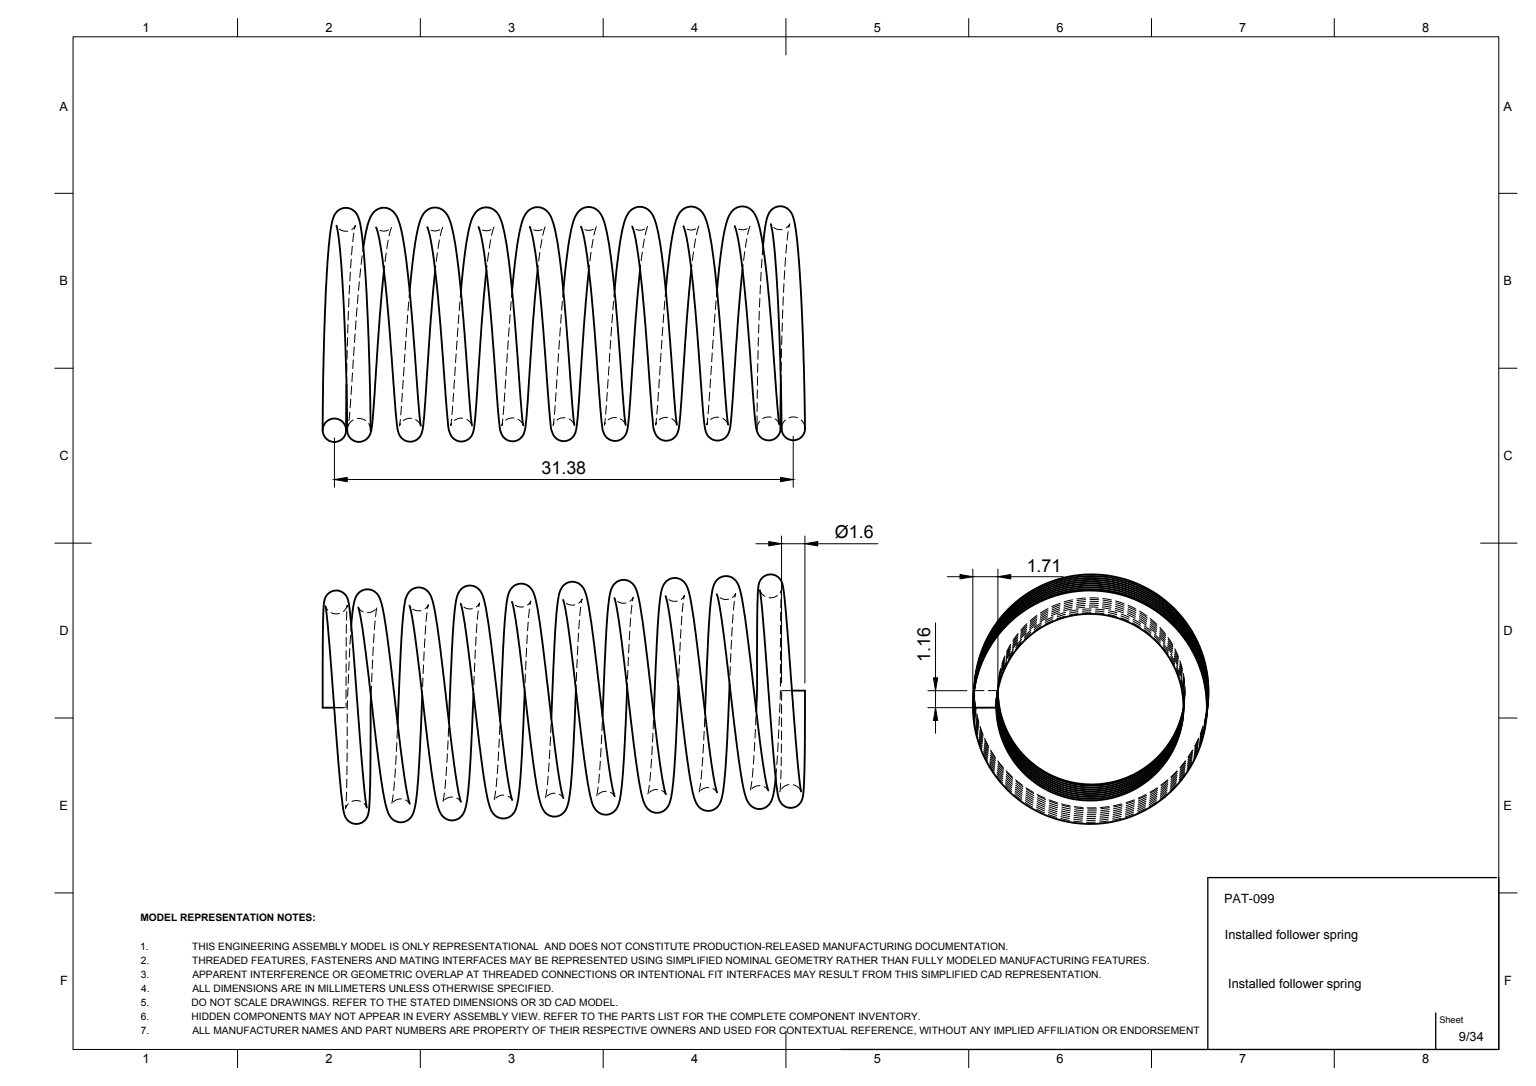
ISO-10303-21;
HEADER;
/* Generated by software containing ST-Developer
 * from STEP Tools, Inc. (www.steptools.com) 
 */

FILE_DESCRIPTION(
/* description */ ('PAT-099'),
/* implementation_level */ '2;1');

FILE_NAME(
/* name */ 'Installed follower spring.step',
/* time_stamp */ '2026-10-29T17:25:42-07:00',
/* author */ (''),
/* organization */ (''),
/* preprocessor_version */ 'ST-DEVELOPER v20.2',
/* originating_system */ 'Autodesk Translation Framework v15.17.0.0',
/* authorisation */ '');

FILE_SCHEMA (('AUTOMOTIVE_DESIGN { 1 0 10303 214 3 1 1 }'));
ENDSEC;

DATA;
#10=MECHANICAL_DESIGN_GEOMETRIC_PRESENTATION_REPRESENTATION('',(#341),#11035);
#240=B_SPLINE_SURFACE_WITH_KNOTS('',3,3,((#7917,#7918,#7919,#7920,#7921,
#7922,#7923,#7924,#7925,#7926,#7927,#7928,#7929,#7930,#7931,#7932,#7933,
#7934,#7935,#7936,#7937,#7938,#7939,#7940,#7941,#7942,#7943,#7944,#7945,
#7946,#7947,#7948,#7949,#7950,#7951,#7952,#7953,#7954,#7955,#7956,#7957,
#7958,#7959,#7960,#7961,#7962,#7963,#7964,#7965,#7966,#7967,#7968,#7969,
#7970,#7971,#7972,#7973,#7974,#7975,#7976,#7977,#7978,#7979,#7980,#7981,
#7982,#7983,#7984,#7985,#7986,#7987,#7988,#7989,#7990,#7991,#7992,#7993,
#7994,#7995,#7996,#7997,#7998,#7999,#8000,#8001,#8002,#8003,#8004,#8005,
#8006,#8007,#8008,#8009,#8010,#8011,#8012,#8013,#8014,#8015,#8016,#8017,
#8018,#8019,#8020,#8021,#8022,#8023,#8024,#8025,#8026,#8027,#8028,#8029,
#8030,#8031,#8032,#8033,#8034,#8035,#8036,#8037,#8038,#8039,#8040,#8041,
#8042,#8043,#8044,#8045,#8046,#8047,#8048,#8049,#8050,#8051,#8052,#8053,
#8054,#8055,#8056),(#8057,#8058,#8059,#8060,#8061,#8062,#8063,#8064,#8065,
#8066,#8067,#8068,#8069,#8070,#8071,#8072,#8073,#8074,#8075,#8076,#8077,
#8078,#8079,#8080,#8081,#8082,#8083,#8084,#8085,#8086,#8087,#8088,#8089,
#8090,#8091,#8092,#8093,#8094,#8095,#8096,#8097,#8098,#8099,#8100,#8101,
#8102,#8103,#8104,#8105,#8106,#8107,#8108,#8109,#8110,#8111,#8112,#8113,
#8114,#8115,#8116,#8117,#8118,#8119,#8120,#8121,#8122,#8123,#8124,#8125,
#8126,#8127,#8128,#8129,#8130,#8131,#8132,#8133,#8134,#8135,#8136,#8137,
#8138,#8139,#8140,#8141,#8142,#8143,#8144,#8145,#8146,#8147,#8148,#8149,
#8150,#8151,#8152,#8153,#8154,#8155,#8156,#8157,#8158,#8159,#8160,#8161,
#8162,#8163,#8164,#8165,#8166,#8167,#8168,#8169,#8170,#8171,#8172,#8173,
#8174,#8175,#8176,#8177,#8178,#8179,#8180,#8181,#8182,#8183,#8184,#8185,
#8186,#8187,#8188,#8189,#8190,#8191,#8192,#8193,#8194,#8195,#8196),(#8197,
#8198,#8199,#8200,#8201,#8202,#8203,#8204,#8205,#8206,#8207,#8208,#8209,
#8210,#8211,#8212,#8213,#8214,#8215,#8216,#8217,#8218,#8219,#8220,#8221,
#8222,#8223,#8224,#8225,#8226,#8227,#8228,#8229,#8230,#8231,#8232,#8233,
#8234,#8235,#8236,#8237,#8238,#8239,#8240,#8241,#8242,#8243,#8244,#8245,
#8246,#8247,#8248,#8249,#8250,#8251,#8252,#8253,#8254,#8255,#8256,#8257,
#8258,#8259,#8260,#8261,#8262,#8263,#8264,#8265,#8266,#8267,#8268,#8269,
#8270,#8271,#8272,#8273,#8274,#8275,#8276,#8277,#8278,#8279,#8280,#8281,
#8282,#8283,#8284,#8285,#8286,#8287,#8288,#8289,#8290,#8291,#8292,#8293,
#8294,#8295,#8296,#8297,#8298,#8299,#8300,#8301,#8302,#8303,#8304,#8305,
#8306,#8307,#8308,#8309,#8310,#8311,#8312,#8313,#8314,#8315,#8316,#8317,
#8318,#8319,#8320,#8321,#8322,#8323,#8324,#8325,#8326,#8327,#8328,#8329,
#8330,#8331,#8332,#8333,#8334,#8335,#8336),(#8337,#8338,#8339,#8340,#8341,
#8342,#8343,#8344,#8345,#8346,#8347,#8348,#8349,#8350,#8351,#8352,#8353,
#8354,#8355,#8356,#8357,#8358,#8359,#8360,#8361,#8362,#8363,#8364,#8365,
#8366,#8367,#8368,#8369,#8370,#8371,#8372,#8373,#8374,#8375,#8376,#8377,
#8378,#8379,#8380,#8381,#8382,#8383,#8384,#8385,#8386,#8387,#8388,#8389,
#8390,#8391,#8392,#8393,#8394,#8395,#8396,#8397,#8398,#8399,#8400,#8401,
#8402,#8403,#8404,#8405,#8406,#8407,#8408,#8409,#8410,#8411,#8412,#8413,
#8414,#8415,#8416,#8417,#8418,#8419,#8420,#8421,#8422,#8423,#8424,#8425,
#8426,#8427,#8428,#8429,#8430,#8431,#8432,#8433,#8434,#8435,#8436,#8437,
#8438,#8439,#8440,#8441,#8442,#8443,#8444,#8445,#8446,#8447,#8448,#8449,
#8450,#8451,#8452,#8453,#8454,#8455,#8456,#8457,#8458,#8459,#8460,#8461,
#8462,#8463,#8464,#8465,#8466,#8467,#8468,#8469,#8470,#8471,#8472,#8473,
#8474,#8475,#8476),(#8477,#8478,#8479,#8480,#8481,#8482,#8483,#8484,#8485,
#8486,#8487,#8488,#8489,#8490,#8491,#8492,#8493,#8494,#8495,#8496,#8497,
#8498,#8499,#8500,#8501,#8502,#8503,#8504,#8505,#8506,#8507,#8508,#8509,
#8510,#8511,#8512,#8513,#8514,#8515,#8516,#8517,#8518,#8519,#8520,#8521,
#8522,#8523,#8524,#8525,#8526,#8527,#8528,#8529,#8530,#8531,#8532,#8533,
#8534,#8535,#8536,#8537,#8538,#8539,#8540,#8541,#8542,#8543,#8544,#8545,
#8546,#8547,#8548,#8549,#8550,#8551,#8552,#8553,#8554,#8555,#8556,#8557,
#8558,#8559,#8560,#8561,#8562,#8563,#8564,#8565,#8566,#8567,#8568,#8569,
#8570,#8571,#8572,#8573,#8574,#8575,#8576,#8577,#8578,#8579,#8580,#8581,
#8582,#8583,#8584,#8585,#8586,#8587,#8588,#8589,#8590,#8591,#8592,#8593,
#8594,#8595,#8596,#8597,#8598,#8599,#8600,#8601,#8602,#8603,#8604,#8605,
#8606,#8607,#8608,#8609,#8610,#8611,#8612,#8613,#8614,#8615,#8616),(#8617,
#8618,#8619,#8620,#8621,#8622,#8623,#8624,#8625,#8626,#8627,#8628,#8629,
#8630,#8631,#8632,#8633,#8634,#8635,#8636,#8637,#8638,#8639,#8640,#8641,
#8642,#8643,#8644,#8645,#8646,#8647,#8648,#8649,#8650,#8651,#8652,#8653,
#8654,#8655,#8656,#8657,#8658,#8659,#8660,#8661,#8662,#8663,#8664,#8665,
#8666,#8667,#8668,#8669,#8670,#8671,#8672,#8673,#8674,#8675,#8676,#8677,
#8678,#8679,#8680,#8681,#8682,#8683,#8684,#8685,#8686,#8687,#8688,#8689,
#8690,#8691,#8692,#8693,#8694,#8695,#8696,#8697,#8698,#8699,#8700,#8701,
#8702,#8703,#8704,#8705,#8706,#8707,#8708,#8709,#8710,#8711,#8712,#8713,
#8714,#8715,#8716,#8717,#8718,#8719,#8720,#8721,#8722,#8723,#8724,#8725,
#8726,#8727,#8728,#8729,#8730,#8731,#8732,#8733,#8734,#8735,#8736,#8737,
#8738,#8739,#8740,#8741,#8742,#8743,#8744,#8745,#8746,#8747,#8748,#8749,
#8750,#8751,#8752,#8753,#8754,#8755,#8756),(#8757,#8758,#8759,#8760,#8761,
#8762,#8763,#8764,#8765,#8766,#8767,#8768,#8769,#8770,#8771,#8772,#8773,
#8774,#8775,#8776,#8777,#8778,#8779,#8780,#8781,#8782,#8783,#8784,#8785,
#8786,#8787,#8788,#8789,#8790,#8791,#8792,#8793,#8794,#8795,#8796,#8797,
#8798,#8799,#8800,#8801,#8802,#8803,#8804,#8805,#8806,#8807,#8808,#8809,
#8810,#8811,#8812,#8813,#8814,#8815,#8816,#8817,#8818,#8819,#8820,#8821,
#8822,#8823,#8824,#8825,#8826,#8827,#8828,#8829,#8830,#8831,#8832,#8833,
#8834,#8835,#8836,#8837,#8838,#8839,#8840,#8841,#8842,#8843,#8844,#8845,
#8846,#8847,#8848,#8849,#8850,#8851,#8852,#8853,#8854,#8855,#8856,#8857,
#8858,#8859,#8860,#8861,#8862,#8863,#8864,#8865,#8866,#8867,#8868,#8869,
#8870,#8871,#8872,#8873,#8874,#8875,#8876,#8877,#8878,#8879,#8880,#8881,
#8882,#8883,#8884,#8885,#8886,#8887,#8888,#8889,#8890,#8891,#8892,#8893,
#8894,#8895,#8896),(#8897,#8898,#8899,#8900,#8901,#8902,#8903,#8904,#8905,
#8906,#8907,#8908,#8909,#8910,#8911,#8912,#8913,#8914,#8915,#8916,#8917,
#8918,#8919,#8920,#8921,#8922,#8923,#8924,#8925,#8926,#8927,#8928,#8929,
#8930,#8931,#8932,#8933,#8934,#8935,#8936,#8937,#8938,#8939,#8940,#8941,
#8942,#8943,#8944,#8945,#8946,#8947,#8948,#8949,#8950,#8951,#8952,#8953,
#8954,#8955,#8956,#8957,#8958,#8959,#8960,#8961,#8962,#8963,#8964,#8965,
#8966,#8967,#8968,#8969,#8970,#8971,#8972,#8973,#8974,#8975,#8976,#8977,
#8978,#8979,#8980,#8981,#8982,#8983,#8984,#8985,#8986,#8987,#8988,#8989,
#8990,#8991,#8992,#8993,#8994,#8995,#8996,#8997,#8998,#8999,#9000,#9001,
#9002,#9003,#9004,#9005,#9006,#9007,#9008,#9009,#9010,#9011,#9012,#9013,
#9014,#9015,#9016,#9017,#9018,#9019,#9020,#9021,#9022,#9023,#9024,#9025,
#9026,#9027,#9028,#9029,#9030,#9031,#9032,#9033,#9034,#9035,#9036),(#9037,
#9038,#9039,#9040,#9041,#9042,#9043,#9044,#9045,#9046,#9047,#9048,#9049,
#9050,#9051,#9052,#9053,#9054,#9055,#9056,#9057,#9058,#9059,#9060,#9061,
#9062,#9063,#9064,#9065,#9066,#9067,#9068,#9069,#9070,#9071,#9072,#9073,
#9074,#9075,#9076,#9077,#9078,#9079,#9080,#9081,#9082,#9083,#9084,#9085,
#9086,#9087,#9088,#9089,#9090,#9091,#9092,#9093,#9094,#9095,#9096,#9097,
#9098,#9099,#9100,#9101,#9102,#9103,#9104,#9105,#9106,#9107,#9108,#9109,
#9110,#9111,#9112,#9113,#9114,#9115,#9116,#9117,#9118,#9119,#9120,#9121,
#9122,#9123,#9124,#9125,#9126,#9127,#9128,#9129,#9130,#9131,#9132,#9133,
#9134,#9135,#9136,#9137,#9138,#9139,#9140,#9141,#9142,#9143,#9144,#9145,
#9146,#9147,#9148,#9149,#9150,#9151,#9152,#9153,#9154,#9155,#9156,#9157,
#9158,#9159,#9160,#9161,#9162,#9163,#9164,#9165,#9166,#9167,#9168,#9169,
#9170,#9171,#9172,#9173,#9174,#9175,#9176),(#9177,#9178,#9179,#9180,#9181,
#9182,#9183,#9184,#9185,#9186,#9187,#9188,#9189,#9190,#9191,#9192,#9193,
#9194,#9195,#9196,#9197,#9198,#9199,#9200,#9201,#9202,#9203,#9204,#9205,
#9206,#9207,#9208,#9209,#9210,#9211,#9212,#9213,#9214,#9215,#9216,#9217,
#9218,#9219,#9220,#9221,#9222,#9223,#9224,#9225,#9226,#9227,#9228,#9229,
#9230,#9231,#9232,#9233,#9234,#9235,#9236,#9237,#9238,#9239,#9240,#9241,
#9242,#9243,#9244,#9245,#9246,#9247,#9248,#9249,#9250,#9251,#9252,#9253,
#9254,#9255,#9256,#9257,#9258,#9259,#9260,#9261,#9262,#9263,#9264,#9265,
#9266,#9267,#9268,#9269,#9270,#9271,#9272,#9273,#9274,#9275,#9276,#9277,
#9278,#9279,#9280,#9281,#9282,#9283,#9284,#9285,#9286,#9287,#9288,#9289,
#9290,#9291,#9292,#9293,#9294,#9295,#9296,#9297,#9298,#9299,#9300,#9301,
#9302,#9303,#9304,#9305,#9306,#9307,#9308,#9309,#9310,#9311,#9312,#9313,
#9314,#9315,#9316)),.UNSPECIFIED.,.T.,.F.,.F.,(4,1,1,1,1,1,1,4),(4,1,1,
1,1,1,1,1,1,1,1,1,1,1,1,1,1,1,1,1,1,1,1,1,1,1,1,1,1,1,1,1,1,1,1,1,1,1,1,
1,1,1,1,1,1,1,1,1,1,1,1,1,1,1,1,1,1,1,1,1,1,1,1,1,1,1,1,1,1,1,1,1,1,1,1,
1,1,1,1,1,1,1,1,1,1,1,1,1,1,1,1,1,1,1,1,1,1,1,1,1,1,1,1,1,1,1,1,1,1,1,1,
1,1,1,1,1,1,1,1,1,1,1,1,1,1,1,1,1,1,1,1,1,1,1,1,1,1,4),(-3.14159265358979,
-2.24399475256414,-1.34639685153848,-0.448798950512828,0.448798950512828,
1.34639685153848,2.24399475256414,3.14159265358979),(0.,0.00892857142857143,
0.0178571428571429,0.0267857142857143,0.0357142857142857,0.0446428571428571,
0.0535714285714286,0.0625,0.0714285714285714,0.0758928571428571,0.0803571428571428,
0.0848214285714286,0.0892857142857143,0.09375,0.0948660714285714,0.0959821428571428,
0.0970982142857143,0.0982142857142857,0.100446428571429,0.102678571428571,
0.107142857142857,0.116071428571429,0.120535714285714,0.125,0.133928571428571,
0.142857142857143,0.150793650793651,0.158730158730159,0.166666666666667,
0.174603174603175,0.182539682539683,0.19047619047619,0.196428571428571,
0.202380952380952,0.214285714285714,0.222222222222222,0.23015873015873,
0.238095238095238,0.241071428571429,0.244047619047619,0.25,0.261904761904762,
0.273809523809524,0.285714285714286,0.297619047619048,0.30952380952381,
0.321428571428571,0.327380952380952,0.333333333333333,0.341269841269841,
0.349206349206349,0.357142857142857,0.361111111111111,0.365079365079365,
0.373015873015873,0.380952380952381,0.392857142857143,0.398809523809524,
0.404761904761905,0.416666666666667,0.428571428571429,0.4375,0.446428571428571,
0.455357142857143,0.457589285714286,0.459821428571429,0.462053571428571,
0.464285714285714,0.470238095238095,0.482142857142857,0.491071428571429,
0.5,0.508928571428571,0.517857142857143,0.526785714285714,0.535714285714286,
0.544642857142857,0.553571428571429,0.5625,0.571428571428571,0.580357142857143,
0.589285714285714,0.598214285714286,0.607142857142857,0.616071428571429,
0.625,0.633928571428571,0.638392857142857,0.642857142857143,0.650793650793651,
0.658730158730159,0.666666666666667,0.672619047619048,0.678571428571428,
0.69047619047619,0.702380952380952,0.714285714285714,0.726190476190476,
0.738095238095238,0.744047619047619,0.75,0.761904761904762,0.76984126984127,
0.777777777777778,0.785714285714286,0.794642857142857,0.803571428571428,
0.8125,0.821428571428571,0.830357142857143,0.839285714285714,0.848214285714286,
0.857142857142857,0.866071428571429,0.875,0.879464285714286,0.883928571428571,
0.892857142857143,0.897321428571428,0.899553571428571,0.901785714285714,
0.902901785714286,0.904017857142857,0.905133928571429,0.90625,0.910714285714286,
0.915178571428571,0.919642857142857,0.924107142857143,0.928571428571429,
0.9375,0.946428571428571,0.955357142857143,0.964285714285714,0.973214285714286,
0.982142857142857,0.991071428571429,1.),.UNSPECIFIED.);
#259=B_SPLINE_CURVE_WITH_KNOTS('',3,(#9320,#9321,#9322,#9323,#9324,#9325,
#9326,#9327,#9328,#9329,#9330,#9331,#9332,#9333,#9334,#9335,#9336,#9337,
#9338,#9339,#9340,#9341,#9342,#9343,#9344,#9345,#9346,#9347,#9348,#9349,
#9350,#9351,#9352,#9353,#9354,#9355,#9356,#9357,#9358,#9359,#9360,#9361,
#9362,#9363,#9364,#9365,#9366,#9367,#9368,#9369,#9370,#9371,#9372,#9373,
#9374,#9375,#9376,#9377,#9378,#9379,#9380,#9381,#9382,#9383,#9384,#9385,
#9386,#9387,#9388,#9389,#9390,#9391,#9392,#9393,#9394,#9395,#9396,#9397,
#9398,#9399,#9400,#9401,#9402,#9403,#9404,#9405,#9406,#9407,#9408,#9409,
#9410,#9411,#9412,#9413,#9414,#9415,#9416,#9417,#9418,#9419,#9420,#9421,
#9422,#9423,#9424,#9425,#9426,#9427,#9428,#9429,#9430,#9431,#9432,#9433,
#9434,#9435,#9436,#9437,#9438,#9439,#9440,#9441,#9442,#9443,#9444,#9445,
#9446,#9447,#9448,#9449,#9450,#9451,#9452,#9453,#9454,#9455,#9456,#9457,
#9458,#9459),.UNSPECIFIED.,.F.,.F.,(4,1,1,1,1,1,1,1,1,1,1,1,1,1,1,1,1,1,
1,1,1,1,1,1,1,1,1,1,1,1,1,1,1,1,1,1,1,1,1,1,1,1,1,1,1,1,1,1,1,1,1,1,1,1,
1,1,1,1,1,1,1,1,1,1,1,1,1,1,1,1,1,1,1,1,1,1,1,1,1,1,1,1,1,1,1,1,1,1,1,1,
1,1,1,1,1,1,1,1,1,1,1,1,1,1,1,1,1,1,1,1,1,1,1,1,1,1,1,1,1,1,1,1,1,1,1,1,
1,1,1,1,1,1,1,1,1,1,1,4),(0.,0.00892857142857143,0.0178571428571429,0.0267857142857143,
0.0357142857142857,0.0446428571428571,0.0535714285714286,0.0625,0.0714285714285714,
0.0758928571428571,0.0803571428571428,0.0848214285714286,0.0892857142857143,
0.09375,0.0948660714285714,0.0959821428571428,0.0970982142857143,0.0982142857142857,
0.100446428571429,0.102678571428571,0.107142857142857,0.116071428571429,
0.120535714285714,0.125,0.133928571428571,0.142857142857143,0.150793650793651,
0.158730158730159,0.166666666666667,0.174603174603175,0.182539682539683,
0.19047619047619,0.196428571428571,0.202380952380952,0.214285714285714,
0.222222222222222,0.23015873015873,0.238095238095238,0.241071428571429,
0.244047619047619,0.25,0.261904761904762,0.273809523809524,0.285714285714286,
0.297619047619048,0.30952380952381,0.321428571428571,0.327380952380952,
0.333333333333333,0.341269841269841,0.349206349206349,0.357142857142857,
0.361111111111111,0.365079365079365,0.373015873015873,0.380952380952381,
0.392857142857143,0.398809523809524,0.404761904761905,0.416666666666667,
0.428571428571429,0.4375,0.446428571428571,0.455357142857143,0.457589285714286,
0.459821428571429,0.462053571428571,0.464285714285714,0.470238095238095,
0.482142857142857,0.491071428571429,0.5,0.508928571428571,0.517857142857143,
0.526785714285714,0.535714285714286,0.544642857142857,0.553571428571429,
0.5625,0.571428571428571,0.580357142857143,0.589285714285714,0.598214285714286,
0.607142857142857,0.616071428571429,0.625,0.633928571428571,0.638392857142857,
0.642857142857143,0.650793650793651,0.658730158730159,0.666666666666667,
0.672619047619048,0.678571428571428,0.69047619047619,0.702380952380952,
0.714285714285714,0.726190476190476,0.738095238095238,0.744047619047619,
0.75,0.761904761904762,0.76984126984127,0.777777777777778,0.785714285714286,
0.794642857142857,0.803571428571428,0.8125,0.821428571428571,0.830357142857143,
0.839285714285714,0.848214285714286,0.857142857142857,0.866071428571429,
0.875,0.879464285714286,0.883928571428571,0.892857142857143,0.897321428571428,
0.899553571428571,0.901785714285714,0.902901785714286,0.904017857142857,
0.905133928571429,0.90625,0.910714285714286,0.915178571428571,0.919642857142857,
0.924107142857143,0.928571428571429,0.9375,0.946428571428571,0.955357142857143,
0.964285714285714,0.973214285714286,0.982142857142857,0.991071428571429,
1.),.UNSPECIFIED.);
#291=SHAPE_REPRESENTATION_RELATIONSHIP('SRR','None',#11159,#316);
#316=ADVANCED_BREP_SHAPE_REPRESENTATION('',(#374),#11009);
#341=STYLED_ITEM('',(#11386),#374);
#374=MANIFOLD_SOLID_BREP('Body1',#4709);
#541=PLANE('',#5146);
#542=PLANE('',#5147);
#714=FACE_OUTER_BOUND('',#1039,.T.);
#715=FACE_OUTER_BOUND('',#1040,.T.);
#716=FACE_OUTER_BOUND('',#1041,.T.);
#1039=EDGE_LOOP('',(#3421,#3422,#3423,#3424));
#1040=EDGE_LOOP('',(#3425));
#1041=EDGE_LOOP('',(#3426));
#1913=CIRCLE('',#5144,0.08);
#1914=CIRCLE('',#5145,0.08);
#2238=VERTEX_POINT('',#9317);
#2239=VERTEX_POINT('',#9319);
#2687=EDGE_CURVE('',#2238,#2238,#1913,.T.);
#2688=EDGE_CURVE('',#2238,#2239,#259,.T.);
#2689=EDGE_CURVE('',#2239,#2239,#1914,.T.);
#3421=ORIENTED_EDGE('',*,*,#2687,.T.);
#3422=ORIENTED_EDGE('',*,*,#2688,.T.);
#3423=ORIENTED_EDGE('',*,*,#2689,.F.);
#3424=ORIENTED_EDGE('',*,*,#2688,.F.);
#3425=ORIENTED_EDGE('',*,*,#2689,.T.);
#3426=ORIENTED_EDGE('',*,*,#2687,.F.);
#4479=ADVANCED_FACE('',(#714),#240,.T.);
#4480=ADVANCED_FACE('',(#715),#541,.T.);
#4481=ADVANCED_FACE('',(#716),#542,.F.);
#4709=CLOSED_SHELL('',(#4479,#4480,#4481));
#5143=AXIS2_PLACEMENT_3D('',#7916,#5983,#5984);
#5144=AXIS2_PLACEMENT_3D('',#9318,#5985,#5986);
#5145=AXIS2_PLACEMENT_3D('',#9460,#5987,#5988);
#5146=AXIS2_PLACEMENT_3D('',#9461,#5989,#5990);
#5147=AXIS2_PLACEMENT_3D('',#9462,#5991,#5992);
#5983=DIRECTION('axis',(0.,0.,1.));
#5984=DIRECTION('refdir',(1.,0.,0.));
#5985=DIRECTION('center_axis',(0.0370000185832032,-0.000134528644531496,
0.999315255826152));
#5986=DIRECTION('ref_axis',(-0.999308650506119,0.00363339380273223,0.0370002631492478));
#5987=DIRECTION('center_axis',(0.0370000189191082,0.000134528641494255,
0.999315255813715));
#5988=DIRECTION('ref_axis',(0.351666218592536,-0.936036645094244,-0.0128945624795743));
#5989=DIRECTION('center_axis',(0.0370000189191082,0.000134528641494255,
0.999315255813715));
#5990=DIRECTION('ref_axis',(0.351666218592536,-0.936036645094244,-0.0128945624795743));
#5991=DIRECTION('center_axis',(0.0370000185832032,-0.000134528644531496,
0.999315255826152));
#5992=DIRECTION('ref_axis',(-0.999308650506119,0.00363339380273222,0.0370002631492478));
#7916=CARTESIAN_POINT('',(0.,0.,0.));
#7917=CARTESIAN_POINT('Ctrl Pts',(6.55994469204049,0.719709328495781,5.24703997894806));
#7918=CARTESIAN_POINT('Ctrl Pts',(6.56494552765653,0.719691145920131,5.38210508200347));
#7919=CARTESIAN_POINT('Ctrl Pts',(6.57494016333875,0.642089168505731,5.65058609468785));
#7920=CARTESIAN_POINT('Ctrl Pts',(6.58989438616266,0.32941528595114,5.9296313569664));
#7921=CARTESIAN_POINT('Ctrl Pts',(6.60481477071411,-0.0827797453005289,
5.99886361370576));
#7922=CARTESIAN_POINT('Ctrl Pts',(6.61969980345594,-0.467619845512657,5.83844773036597));
#7923=CARTESIAN_POINT('Ctrl Pts',(6.63454965842308,-0.707639327219362,5.49857002500469));
#7924=CARTESIAN_POINT('Ctrl Pts',(6.64936061260475,-0.729495436544756,5.0840660001111));
#7925=CARTESIAN_POINT('Ctrl Pts',(6.66414030226907,-0.527844751315962,4.72224444577032));
#7926=CARTESIAN_POINT('Ctrl Pts',(6.67641810037933,-0.225796647591973,4.55722222010489));
#7927=CARTESIAN_POINT('Ctrl Pts',(6.68623494447203,0.0403746271135037,4.5362580751361));
#7928=CARTESIAN_POINT('Ctrl Pts',(6.69357256905876,0.236291461979514,4.57606849800983));
#7929=CARTESIAN_POINT('Ctrl Pts',(6.70093718034598,0.413303779793928,4.66864974641035));
#7930=CARTESIAN_POINT('Ctrl Pts',(6.70820868996388,0.557592736564421,4.80642809587619));
#7931=CARTESIAN_POINT('Ctrl Pts',(6.71380490830661,0.632807795501951,4.93556873282767));
#7932=CARTESIAN_POINT('Ctrl Pts',(6.71731244248601,0.666836920456702,5.02812885948168));
#7933=CARTESIAN_POINT('Ctrl Pts',(6.71917582310349,0.680406120596861,5.07513188532028));
#7934=CARTESIAN_POINT('Ctrl Pts',(6.72133213271133,0.6909093875254,5.1233938812218));
#7935=CARTESIAN_POINT('Ctrl Pts',(6.72306773259333,0.700241175081311,5.19054637990825));
#7936=CARTESIAN_POINT('Ctrl Pts',(6.72619261442483,0.703178325652587,5.2668476785023));
#7937=CARTESIAN_POINT('Ctrl Pts',(6.7381664251681,0.689514001675121,5.39852659753196));
#7938=CARTESIAN_POINT('Ctrl Pts',(6.75463925550615,0.618247264838858,5.61826960075177));
#7939=CARTESIAN_POINT('Ctrl Pts',(6.77590827674278,0.436470460186145,5.81941560675087));
#7940=CARTESIAN_POINT('Ctrl Pts',(6.79564326301645,0.196280809931693,5.9247163591309));
#7941=CARTESIAN_POINT('Ctrl Pts',(6.81582644522033,-0.0629302930494358,
5.96025522192144));
#7942=CARTESIAN_POINT('Ctrl Pts',(6.84069654900574,-0.38497400844017,5.86555713916006));
#7943=CARTESIAN_POINT('Ctrl Pts',(6.86947638412051,-0.640427331596973,5.57601421543896));
#7944=CARTESIAN_POINT('Ctrl Pts',(6.89697365083529,-0.710923798883682,5.21615884811777));
#7945=CARTESIAN_POINT('Ctrl Pts',(6.92329898795441,-0.605777386429107,4.88177837844538));
#7946=CARTESIAN_POINT('Ctrl Pts',(6.94951107797999,-0.354456178032768,4.63917675459059));
#7947=CARTESIAN_POINT('Ctrl Pts',(6.97563701108018,-0.0190898795841548,
4.54673256040166));
#7948=CARTESIAN_POINT('Ctrl Pts',(7.00166306815893,0.318420157020357,4.6254869521555));
#7949=CARTESIAN_POINT('Ctrl Pts',(7.02543388521809,0.554722542828515,4.83645416115326));
#7950=CARTESIAN_POINT('Ctrl Pts',(7.04697773806416,0.666084600719225,5.09617679024369));
#7951=CARTESIAN_POINT('Ctrl Pts',(7.07276315353201,0.678427725557665,5.43526847721852));
#7952=CARTESIAN_POINT('Ctrl Pts',(7.10058962059944,0.484472501752673,5.76690932949108));
#7953=CARTESIAN_POINT('Ctrl Pts',(7.13043692169364,0.120638399689201,5.92825455906627));
#7954=CARTESIAN_POINT('Ctrl Pts',(7.1559402685194,-0.217537459809761,5.90145833585114));
#7955=CARTESIAN_POINT('Ctrl Pts',(7.17606991375773,-0.442156866353605,5.75500273582888));
#7956=CARTESIAN_POINT('Ctrl Pts',(7.1908732639631,-0.55830610816236,5.60220615030058));
#7957=CARTESIAN_POINT('Ctrl Pts',(7.20354845498638,-0.631705810891337,5.45532626907927));
#7958=CARTESIAN_POINT('Ctrl Pts',(7.22569553162755,-0.685810607871027,5.1691057765553));
#7959=CARTESIAN_POINT('Ctrl Pts',(7.25723947880328,-0.525122526582691,4.7636055764722));
#7960=CARTESIAN_POINT('Ctrl Pts',(7.29495362238925,-0.053457135933399,4.53870854204931));
#7961=CARTESIAN_POINT('Ctrl Pts',(7.33254246780218,0.443142598581714,4.69413693222259));
#7962=CARTESIAN_POINT('Ctrl Pts',(7.37001978026861,0.701091243696442,5.14423427781829));
#7963=CARTESIAN_POINT('Ctrl Pts',(7.40739968824424,0.584157721738047,5.64880921553006));
#7964=CARTESIAN_POINT('Ctrl Pts',(7.43848048896546,0.228011772623945,5.88938664283398));
#7965=CARTESIAN_POINT('Ctrl Pts',(7.46331103237168,-0.0982454758707846,
5.89962806423389));
#7966=CARTESIAN_POINT('Ctrl Pts',(7.48398628613683,-0.354294590444537,5.80983193950292));
#7967=CARTESIAN_POINT('Ctrl Pts',(7.50671008387199,-0.570451156260486,5.59791253961241));
#7968=CARTESIAN_POINT('Ctrl Pts',(7.53148051029953,-0.667000675030891,5.28247942808214));
#7969=CARTESIAN_POINT('Ctrl Pts',(7.55211030997723,-0.61172699107091,5.01340213779963));
#7970=CARTESIAN_POINT('Ctrl Pts',(7.56860908294787,-0.494743373007304,4.8335093105102));
#7971=CARTESIAN_POINT('Ctrl Pts',(7.58510523358743,-0.337168872759663,4.68756299395369));
#7972=CARTESIAN_POINT('Ctrl Pts',(7.60572192687897,-0.0819019612031444,
4.58805237352457));
#7973=CARTESIAN_POINT('Ctrl Pts',(7.63458408889819,0.300170619986696,4.63555033917682));
#7974=CARTESIAN_POINT('Ctrl Pts',(7.66138943476793,0.571053603076512,4.88796924826266));
#7975=CARTESIAN_POINT('Ctrl Pts',(7.68614446458683,0.653366892065435,5.20295921197447));
#7976=CARTESIAN_POINT('Ctrl Pts',(7.71090979818012,0.617991353788974,5.52603673989692));
#7977=CARTESIAN_POINT('Ctrl Pts',(7.74189055099461,0.350623503322525,5.86154592695952));
#7978=CARTESIAN_POINT('Ctrl Pts',(7.77601859800523,-0.116495965826188,5.93082813098408));
#7979=CARTESIAN_POINT('Ctrl Pts',(7.80709414997369,-0.481412412605556,5.72789933690448));
#7980=CARTESIAN_POINT('Ctrl Pts',(7.83510698559819,-0.663163478596285,5.39892523906655));
#7981=CARTESIAN_POINT('Ctrl Pts',(7.85615485977222,-0.647079306054213,5.11675578479515));
#7982=CARTESIAN_POINT('Ctrl Pts',(7.87020459706828,-0.574886104874813,4.94990033899215));
#7983=CARTESIAN_POINT('Ctrl Pts',(7.87723312367712,-0.527583060020924,4.87226677612988));
#7984=CARTESIAN_POINT('Ctrl Pts',(7.88426540124521,-0.469793796464868,4.80191051673322));
#7985=CARTESIAN_POINT('Ctrl Pts',(7.89521047892777,-0.365529336701908,4.7063343213378));
#7986=CARTESIAN_POINT('Ctrl Pts',(7.91634048666751,-0.120063962380262,4.57508935662309));
#7987=CARTESIAN_POINT('Ctrl Pts',(7.94458071734118,0.268642859242054,4.60441791433467));
#7988=CARTESIAN_POINT('Ctrl Pts',(7.97605533596052,0.584027938453731,4.88737223927164));
#7989=CARTESIAN_POINT('Ctrl Pts',(8.00446254702578,0.689638060716412,5.2531749302134));
#7990=CARTESIAN_POINT('Ctrl Pts',(8.03295521872146,0.583958260807566,5.62109535966095));
#7991=CARTESIAN_POINT('Ctrl Pts',(8.06153860386915,0.297951770638925,5.87686527268886));
#7992=CARTESIAN_POINT('Ctrl Pts',(8.09021776831132,-0.0816004700383042,
5.94171985993802));
#7993=CARTESIAN_POINT('Ctrl Pts',(8.11899761019108,-0.438736741574054,5.7941606881638));
#7994=CARTESIAN_POINT('Ctrl Pts',(8.14788283876726,-0.66350439566471,5.47812772009615));
#7995=CARTESIAN_POINT('Ctrl Pts',(8.17687795851733,-0.6858207744463,5.08946678694388));
#7996=CARTESIAN_POINT('Ctrl Pts',(8.20598727446933,-0.497249207778955,4.74714184053921));
#7997=CARTESIAN_POINT('Ctrl Pts',(8.23521486961617,-0.154093127286878,4.55679071733693));
#7998=CARTESIAN_POINT('Ctrl Pts',(8.26456461818433,0.239380388009074,4.57821827016813));
#7999=CARTESIAN_POINT('Ctrl Pts',(8.29404014876887,0.562549974717286,4.80663318942082));
#8000=CARTESIAN_POINT('Ctrl Pts',(8.32364486518472,0.715391021033525,5.17354565176085));
#8001=CARTESIAN_POINT('Ctrl Pts',(8.35338192623768,0.649330974858417,5.56731319891309));
#8002=CARTESIAN_POINT('Ctrl Pts',(8.38325424070601,0.382790348017333,5.86693311075399));
#8003=CARTESIAN_POINT('Ctrl Pts',(8.41326446409716,-0.00419505000370753,
5.97947359705855));
#8004=CARTESIAN_POINT('Ctrl Pts',(8.43838990507217,-0.328427739096548,5.88675138216907));
#8005=CARTESIAN_POINT('Ctrl Pts',(8.45856147729175,-0.529480619639225,5.71722997945441));
#8006=CARTESIAN_POINT('Ctrl Pts',(8.47765754585014,-0.668434606896997,5.5107649981822));
#8007=CARTESIAN_POINT('Ctrl Pts',(8.50076123794206,-0.730336170493974,5.20937619755011));
#8008=CARTESIAN_POINT('Ctrl Pts',(8.52792461605616,-0.624513035959022,4.86362366838459));
#8009=CARTESIAN_POINT('Ctrl Pts',(8.5529308052989,-0.386883838373545,4.6302289824672));
#8010=CARTESIAN_POINT('Ctrl Pts',(8.57574894485481,-0.104298108040022,4.53121501380808));
#8011=CARTESIAN_POINT('Ctrl Pts',(8.6032187287894,0.256675810750089,4.54226136093568));
#8012=CARTESIAN_POINT('Ctrl Pts',(8.63772155686955,0.652405168310869,4.80876975888547));
#8013=CARTESIAN_POINT('Ctrl Pts',(8.67939097890975,0.783030401351032,5.37140034010679));
#8014=CARTESIAN_POINT('Ctrl Pts',(8.72132656843746,0.49495090614558,5.87513455402037));
#8015=CARTESIAN_POINT('Ctrl Pts',(8.76352759225084,-0.0628635021467805,
6.05013777316939));
#8016=CARTESIAN_POINT('Ctrl Pts',(8.79891493140875,-0.504716359285686,5.83905645697925));
#8017=CARTESIAN_POINT('Ctrl Pts',(8.82735545219243,-0.703159459402567,5.5227896978014));
#8018=CARTESIAN_POINT('Ctrl Pts',(8.85588259535385,-0.776061781005718,5.15482469233793));
#8019=CARTESIAN_POINT('Ctrl Pts',(8.88692644387892,-0.621492770362474,4.75483748689365));
#8020=CARTESIAN_POINT('Ctrl Pts',(8.92052297991862,-0.245496738926199,4.51104937209089));
#8021=CARTESIAN_POINT('Ctrl Pts',(8.94943095663315,0.137693585331708,4.48033145317999));
#8022=CARTESIAN_POINT('Ctrl Pts',(8.97965767299615,0.505669735297425,4.64426980471776));
#8023=CARTESIAN_POINT('Ctrl Pts',(9.01121604967911,0.752482582266742,4.98850418901732));
#8024=CARTESIAN_POINT('Ctrl Pts',(9.04412144632782,0.779510405814253,5.42959222113123));
#8025=CARTESIAN_POINT('Ctrl Pts',(9.07715711994043,0.566889248726445,5.81885947968755));
#8026=CARTESIAN_POINT('Ctrl Pts',(9.11031735538565,0.178292209075846,6.0362617860296));
#8027=CARTESIAN_POINT('Ctrl Pts',(9.14360253722173,-0.268079437778697,6.01351727669282));
#8028=CARTESIAN_POINT('Ctrl Pts',(9.17699734546285,-0.635285771434068,5.75590592911153));
#8029=CARTESIAN_POINT('Ctrl Pts',(9.21051983173094,-0.809796215592389,5.34095865996421));
#8030=CARTESIAN_POINT('Ctrl Pts',(9.24411094986739,-0.736619369561702,4.89534022537719));
#8031=CARTESIAN_POINT('Ctrl Pts',(9.27788074499435,-0.436616793358521,4.55570108560577));
#8032=CARTESIAN_POINT('Ctrl Pts',(9.30594116368128,-0.0733420592947115,
4.44897069772665));
#8033=CARTESIAN_POINT('Ctrl Pts',(9.328680473888,0.218704827060702,4.48901682699427));
#8034=CARTESIAN_POINT('Ctrl Pts',(9.35089495840618,0.489065381509997,4.60762593183536));
#8035=CARTESIAN_POINT('Ctrl Pts',(9.37480209610635,0.693278005812641,4.83358316838714));
#8036=CARTESIAN_POINT('Ctrl Pts',(9.39327740184756,0.773205179450414,5.08031011736591));
#8037=CARTESIAN_POINT('Ctrl Pts',(9.40667901531909,0.788514168138214,5.22730031946394));
#8038=CARTESIAN_POINT('Ctrl Pts',(9.41035265957923,0.785191918284243,5.31605807341251));
#8039=CARTESIAN_POINT('Ctrl Pts',(9.41223809751033,0.774762970480976,5.39019446309586));
#8040=CARTESIAN_POINT('Ctrl Pts',(9.4146591021466,0.763068583364469,5.44423938068532));
#8041=CARTESIAN_POINT('Ctrl Pts',(9.4167523666832,0.747778571803171,5.49710428778674));
#8042=CARTESIAN_POINT('Ctrl Pts',(9.42068446598339,0.709658392601865,5.60083098220104));
#8043=CARTESIAN_POINT('Ctrl Pts',(9.42695148511213,0.625399217361514,5.74546397737963));
#8044=CARTESIAN_POINT('Ctrl Pts',(9.4350913459169,0.463897848898915,5.89967743034001));
#8045=CARTESIAN_POINT('Ctrl Pts',(9.44332988824765,0.265871334396363,6.00323600320908));
#8046=CARTESIAN_POINT('Ctrl Pts',(9.45153347644623,0.0468430344411857,6.04773546710682));
#8047=CARTESIAN_POINT('Ctrl Pts',(9.46250188685132,-0.250556076226033,6.02429177474909));
#8048=CARTESIAN_POINT('Ctrl Pts',(9.47620737800529,-0.587650060167328,5.84004639330421));
#8049=CARTESIAN_POINT('Ctrl Pts',(9.49268366719886,-0.81241635296479,5.43659555942134));
#8050=CARTESIAN_POINT('Ctrl Pts',(9.50917374900608,-0.787865415172378,4.9752477474741));
#8051=CARTESIAN_POINT('Ctrl Pts',(9.52568233488031,-0.521201295938573,4.59717415541696));
#8052=CARTESIAN_POINT('Ctrl Pts',(9.5422061736552,-0.0937383220535699,4.41946428983354));
#8053=CARTESIAN_POINT('Ctrl Pts',(9.55874735915243,0.363109547604185,4.49620059730279));
#8054=CARTESIAN_POINT('Ctrl Pts',(9.57529830568314,0.709172657538417,4.80516325810888));
#8055=CARTESIAN_POINT('Ctrl Pts',(9.58634758255215,0.794862864598598,5.10196837702893));
#8056=CARTESIAN_POINT('Ctrl Pts',(9.59186670251247,0.79488293160754,5.25103156499837));
#8057=CARTESIAN_POINT('Ctrl Pts',(6.5600317203433,0.743645114310226,5.24703997894806));
#8058=CARTESIAN_POINT('Ctrl Pts',(6.56519694359966,0.743626334036324,5.38654494671483));
#8059=CARTESIAN_POINT('Ctrl Pts',(6.57552575104629,0.663439491064011,5.66398423458453));
#8060=CARTESIAN_POINT('Ctrl Pts',(6.59097732705008,0.340362727022784,5.95229610571387));
#8061=CARTESIAN_POINT('Ctrl Pts',(6.60639588256248,-0.085564624808665,6.02384672671786));
#8062=CARTESIAN_POINT('Ctrl Pts',(6.62177750449655,-0.483232072698951,5.85808296752321));
#8063=CARTESIAN_POINT('Ctrl Pts',(6.63712358115281,-0.73125343445,5.50687494047551));
#8064=CARTESIAN_POINT('Ctrl Pts',(6.65243043600796,-0.753834594795398,5.07854546230159));
#8065=CARTESIAN_POINT('Ctrl Pts',(6.6677040836227,-0.545458428391592,4.70466776269486));
#8066=CARTESIAN_POINT('Ctrl Pts',(6.68039282388046,-0.23334272044992,4.53415317767454));
#8067=CARTESIAN_POINT('Ctrl Pts',(6.69053665092139,0.0416796042804993,4.51249422389647));
#8068=CARTESIAN_POINT('Ctrl Pts',(6.69811867522059,0.244107755344965,4.55362929691641));
#8069=CARTESIAN_POINT('Ctrl Pts',(6.70572848762197,0.426997624599347,4.64928698265267));
#8070=CARTESIAN_POINT('Ctrl Pts',(6.713241694215,0.576073511958108,4.79163606897931));
#8071=CARTESIAN_POINT('Ctrl Pts',(6.71902424219905,0.653781708136255,4.92505878976939));
#8072=CARTESIAN_POINT('Ctrl Pts',(6.72264773696813,0.688937202960286,5.0206791373597));
#8073=CARTESIAN_POINT('Ctrl Pts',(6.72457239960857,0.702948690130069,5.069221824819));
#8074=CARTESIAN_POINT('Ctrl Pts',(6.72679968927165,0.713804995118134,5.1190819534982));
#8075=CARTESIAN_POINT('Ctrl Pts',(6.7285973777106,0.723447631782051,5.18854189286989));
#8076=CARTESIAN_POINT('Ctrl Pts',(6.73181253270818,0.726479171259777,5.26711526304695));
#8077=CARTESIAN_POINT('Ctrl Pts',(6.74418104973988,0.712364538955456,5.40315993041796));
#8078=CARTESIAN_POINT('Ctrl Pts',(6.76119416892908,0.638762136278474,5.63009066315064));
#8079=CARTESIAN_POINT('Ctrl Pts',(6.78316216266072,0.451029028315658,5.83780909913891));
#8080=CARTESIAN_POINT('Ctrl Pts',(6.80353597647317,0.203074911136787,5.94650492858841));
#8081=CARTESIAN_POINT('Ctrl Pts',(6.8243697854844,-0.0644746999694365,5.98318447082224));
#8082=CARTESIAN_POINT('Ctrl Pts',(6.85003803144352,-0.396790077585058,5.885439852334));
#8083=CARTESIAN_POINT('Ctrl Pts',(6.8797274902126,-0.660254447903026,5.586770643378));
#8084=CARTESIAN_POINT('Ctrl Pts',(6.90808044479718,-0.732907685022115,5.21576889406585));
#8085=CARTESIAN_POINT('Ctrl Pts',(6.93521165231085,-0.624533500927869,4.87121325841169));
#8086=CARTESIAN_POINT('Ctrl Pts',(6.96221299448147,-0.365673416845925,4.62137630968268));
#8087=CARTESIAN_POINT('Ctrl Pts',(6.98910503562642,-0.0204912870103402,
4.52625933591179));
#8088=CARTESIAN_POINT('Ctrl Pts',(7.01587828254526,0.326664127736654,4.60729823930461));
#8089=CARTESIAN_POINT('Ctrl Pts',(7.04031755717951,0.569540378656345,4.82418452570712));
#8090=CARTESIAN_POINT('Ctrl Pts',(7.06244951669149,0.683917755846529,5.09097740656128));
#8091=CARTESIAN_POINT('Ctrl Pts',(7.08892444932795,0.696562702579088,5.43910230418443));
#8092=CARTESIAN_POINT('Ctrl Pts',(7.11747479399797,0.497535769821888,5.77923828692686));
#8093=CARTESIAN_POINT('Ctrl Pts',(7.14805659228038,0.12476158764217,5.9444858162509));
#8094=CARTESIAN_POINT('Ctrl Pts',(7.17416577049173,-0.221392458573116,5.91702498690739));
#8095=CARTESIAN_POINT('Ctrl Pts',(7.19475934143304,-0.451091723068877,5.76721176820514));
#8096=CARTESIAN_POINT('Ctrl Pts',(7.20988756684039,-0.569776469467092,5.6110768737848));
#8097=CARTESIAN_POINT('Ctrl Pts',(7.22283668157726,-0.644749444213715,5.46104198585997));
#8098=CARTESIAN_POINT('Ctrl Pts',(7.2454490573998,-0.699961029561219,5.16883668420344));
#8099=CARTESIAN_POINT('Ctrl Pts',(7.27762148574156,-0.535981776011502,4.75540507774079));
#8100=CARTESIAN_POINT('Ctrl Pts',(7.31601994074765,-0.0557826574189054,
4.52663770463754));
#8101=CARTESIAN_POINT('Ctrl Pts',(7.354222969087,0.448762644999277,4.68474223075386));
#8102=CARTESIAN_POINT('Ctrl Pts',(7.39224226780421,0.710217511679504,5.14133781559877));
#8103=CARTESIAN_POINT('Ctrl Pts',(7.43008902366988,0.5916594052894,5.65206211899789));
#8104=CARTESIAN_POINT('Ctrl Pts',(7.4614980372404,0.231764021629228,5.89497907260121));
#8105=CARTESIAN_POINT('Ctrl Pts',(7.48654869737898,-0.0973240615553253,
5.9052786006524));
#8106=CARTESIAN_POINT('Ctrl Pts',(7.50738456391928,-0.355323659444364,5.81476648546977));
#8107=CARTESIAN_POINT('Ctrl Pts',(7.53026554544261,-0.572856338749848,5.60142020877485));
#8108=CARTESIAN_POINT('Ctrl Pts',(7.55517056925149,-0.669836218441959,5.28435098152571));
#8109=CARTESIAN_POINT('Ctrl Pts',(7.57588102694464,-0.614317827947794,5.01429935338668));
#8110=CARTESIAN_POINT('Ctrl Pts',(7.59242404307814,-0.497025790221269,4.83395433811505));
#8111=CARTESIAN_POINT('Ctrl Pts',(7.6089536687432,-0.339149431178674,4.68774659297558));
#8112=CARTESIAN_POINT('Ctrl Pts',(7.62959668968493,-0.0836344771110079,
4.58817926603548));
#8113=CARTESIAN_POINT('Ctrl Pts',(7.65844010764145,0.298170598732022,4.63573436796571));
#8114=CARTESIAN_POINT('Ctrl Pts',(7.68518935302475,0.568322726393191,4.88764401261463));
#8115=CARTESIAN_POINT('Ctrl Pts',(7.70984650366045,0.650261419625715,5.20136259590943));
#8116=CARTESIAN_POINT('Ctrl Pts',(7.7344907134544,0.615036584967239,5.5228070000813));
#8117=CARTESIAN_POINT('Ctrl Pts',(7.76527474802387,0.349308839296457,5.8559972266997));
#8118=CARTESIAN_POINT('Ctrl Pts',(7.79911144782391,-0.113753064206836,5.92449976127185));
#8119=CARTESIAN_POINT('Ctrl Pts',(7.82986619410816,-0.474773880924156,5.72362564992567));
#8120=CARTESIAN_POINT('Ctrl Pts',(7.85755227579443,-0.654292059961964,5.39855675400986));
#8121=CARTESIAN_POINT('Ctrl Pts',(7.87832541447077,-0.638370401196948,5.12017204060674));
#8122=CARTESIAN_POINT('Ctrl Pts',(7.89217334819649,-0.567221155458292,4.95572879884478));
#8123=CARTESIAN_POINT('Ctrl Pts',(7.89909834733727,-0.520617423747659,4.87924437693166));
#8124=CARTESIAN_POINT('Ctrl Pts',(7.90602450006169,-0.46370339051325,4.80995566767418));
#8125=CARTESIAN_POINT('Ctrl Pts',(7.91680097396861,-0.361054204005317,4.71586067278074));
#8126=CARTESIAN_POINT('Ctrl Pts',(7.93759389399371,-0.119518166224153,4.58675402992836));
#8127=CARTESIAN_POINT('Ctrl Pts',(7.96534006210386,0.26236475600673,4.61568621451773));
#8128=CARTESIAN_POINT('Ctrl Pts',(7.99622107554029,0.571693519917959,4.89331989674528));
#8129=CARTESIAN_POINT('Ctrl Pts',(8.02405932467958,0.675115995227338,5.25172945407709));
#8130=CARTESIAN_POINT('Ctrl Pts',(8.05194395308582,0.571652421174932,5.61172186136834));
#8131=CARTESIAN_POINT('Ctrl Pts',(8.07988411081677,0.292101156534909,5.86164971137292));
#8132=CARTESIAN_POINT('Ctrl Pts',(8.10788501784531,-0.0784233387711395,
5.92490818089582));
#8133=CARTESIAN_POINT('Ctrl Pts',(8.13595344261398,-0.426656560206351,5.78097145446324));
#8134=CARTESIAN_POINT('Ctrl Pts',(8.16409525054265,-0.645567978861292,5.47308673944232));
#8135=CARTESIAN_POINT('Ctrl Pts',(8.19231648013073,-0.667238707993714,5.09484527058636));
#8136=CARTESIAN_POINT('Ctrl Pts',(8.22062287004232,-0.483851359843703,4.76202254371853));
#8137=CARTESIAN_POINT('Ctrl Pts',(8.24902004521049,-0.150460572151325,4.57713441531565));
#8138=CARTESIAN_POINT('Ctrl Pts',(8.27751345201596,0.231494106069571,4.59797138762446));
#8139=CARTESIAN_POINT('Ctrl Pts',(8.30610832696761,0.544962336065687,4.81956979365873));
#8140=CARTESIAN_POINT('Ctrl Pts',(8.33480976434835,0.69310132607455,5.17527118660301));
#8141=CARTESIAN_POINT('Ctrl Pts',(8.36362257168318,0.629073409022718,5.55677031488762));
#8142=CARTESIAN_POINT('Ctrl Pts',(8.3925515424265,0.370948750229092,5.84689628452807));
#8143=CARTESIAN_POINT('Ctrl Pts',(8.42160081890503,-0.00363259840954581,
5.95581045784778));
#8144=CARTESIAN_POINT('Ctrl Pts',(8.44591291482813,-0.317350461105933,5.86608437702079));
#8145=CARTESIAN_POINT('Ctrl Pts',(8.46542612591725,-0.511837377716034,5.70209791662713));
#8146=CARTESIAN_POINT('Ctrl Pts',(8.48389640313918,-0.646235426932618,5.50240070801776));
#8147=CARTESIAN_POINT('Ctrl Pts',(8.50623968962513,-0.706096395161048,5.21093606001156));
#8148=CARTESIAN_POINT('Ctrl Pts',(8.5325044635867,-0.603771630310612,4.87662564951356));
#8149=CARTESIAN_POINT('Ctrl Pts',(8.55668059344481,-0.374029117623404,4.65097664338371));
#8150=CARTESIAN_POINT('Ctrl Pts',(8.5787403647823,-0.100834246650297,4.555251023442));
#8151=CARTESIAN_POINT('Ctrl Pts',(8.60529688102436,0.248141502636759,4.56592896275675));
#8152=CARTESIAN_POINT('Ctrl Pts',(8.63865284797812,0.63073545090754,4.82357537459606));
#8153=CARTESIAN_POINT('Ctrl Pts',(8.67894294821516,0.757069626679118,5.36759646206742));
#8154=CARTESIAN_POINT('Ctrl Pts',(8.71950063159077,0.478476625654173,5.85482636408642));
#8155=CARTESIAN_POINT('Ctrl Pts',(8.76033010054568,-0.0612231371037712,
6.0242021516719));
#8156=CARTESIAN_POINT('Ctrl Pts',(8.79458253319758,-0.488965462755427,5.81992360842052));
#8157=CARTESIAN_POINT('Ctrl Pts',(8.82212390948946,-0.681160794137239,5.5136406662995));
#8158=CARTESIAN_POINT('Ctrl Pts',(8.84975893027925,-0.751796896761062,5.1571792721246));
#8159=CARTESIAN_POINT('Ctrl Pts',(8.87984444837189,-0.602041078690657,4.76948039106712));
#8160=CARTESIAN_POINT('Ctrl Pts',(8.91242785081629,-0.237384194390308,4.53301014325183));
#8161=CARTESIAN_POINT('Ctrl Pts',(8.94047881699228,0.134466585038931,4.50317155345517));
#8162=CARTESIAN_POINT('Ctrl Pts',(8.96982711252411,0.491781010059867,4.66232849803431));
#8163=CARTESIAN_POINT('Ctrl Pts',(9.00048403532161,0.731620029022094,4.99675916496741));
#8164=CARTESIAN_POINT('Ctrl Pts',(9.03247511104355,0.75794664861164,5.42565043938059));
#8165=CARTESIAN_POINT('Ctrl Pts',(9.06461825742226,0.551078368819278,5.80448348845649));
#8166=CARTESIAN_POINT('Ctrl Pts',(9.09690994076132,0.172623636920341,6.01627057338027));
#8167=CARTESIAN_POINT('Ctrl Pts',(9.12935177960436,-0.262514946567701,5.99415428011165));
#8168=CARTESIAN_POINT('Ctrl Pts',(9.16193014094924,-0.620844213656014,5.74284535005782));
#8169=CARTESIAN_POINT('Ctrl Pts',(9.19466437324471,-0.791343274428717,5.33760912799968));
#8170=CARTESIAN_POINT('Ctrl Pts',(9.22749713604095,-0.719879593774102,4.90194850755568));
#8171=CARTESIAN_POINT('Ctrl Pts',(9.26053924327341,-0.426350462849809,4.56952461792616));
#8172=CARTESIAN_POINT('Ctrl Pts',(9.2880208954263,-0.0705095289102926,4.46489634881681));
#8173=CARTESIAN_POINT('Ctrl Pts',(9.31031394458354,0.215835839245267,4.50415210664416));
#8174=CARTESIAN_POINT('Ctrl Pts',(9.33210485242398,0.481055339319739,4.62046584167929));
#8175=CARTESIAN_POINT('Ctrl Pts',(9.35556651022956,0.681566722795924,4.84232209585076));
#8176=CARTESIAN_POINT('Ctrl Pts',(9.37372634427259,0.76013142053573,5.0847068874864));
#8177=CARTESIAN_POINT('Ctrl Pts',(9.38691189586978,0.775186012058393,5.22951776549698));
#8178=CARTESIAN_POINT('Ctrl Pts',(9.39044111391715,0.771934376682021,5.31522516777114));
#8179=CARTESIAN_POINT('Ctrl Pts',(9.39232430774748,0.761663575933829,5.38868371146561));
#8180=CARTESIAN_POINT('Ctrl Pts',(9.39470301848468,0.750125538816929,5.44185526499922));
#8181=CARTESIAN_POINT('Ctrl Pts',(9.39675915672847,0.735128865991617,5.4937547021154));
#8182=CARTESIAN_POINT('Ctrl Pts',(9.40062547913648,0.697631703938273,5.59576957012101));
#8183=CARTESIAN_POINT('Ctrl Pts',(9.40678906395115,0.614761668799333,5.73804352075162));
#8184=CARTESIAN_POINT('Ctrl Pts',(9.41479721859882,0.455844412061066,5.88979323730855));
#8185=CARTESIAN_POINT('Ctrl Pts',(9.42290476320863,0.260938548878604,5.99172438224085));
#8186=CARTESIAN_POINT('Ctrl Pts',(9.43098028733991,0.0452935297457695,6.03554040196323));
#8187=CARTESIAN_POINT('Ctrl Pts',(9.44178112627354,-0.24759975779143,6.01245735507339));
#8188=CARTESIAN_POINT('Ctrl Pts',(9.45527918626336,-0.579717863548197,5.83096339648743));
#8189=CARTESIAN_POINT('Ctrl Pts',(9.47151748582056,-0.801334910259173,5.43325751280776));
#8190=CARTESIAN_POINT('Ctrl Pts',(9.48777877066663,-0.777156535330782,4.97819185288487));
#8191=CARTESIAN_POINT('Ctrl Pts',(9.50406651147499,-0.514028895195191,4.60503104228514));
#8192=CARTESIAN_POINT('Ctrl Pts',(9.52038183374562,-0.0919082290386587,
4.42949936533505));
#8193=CARTESIAN_POINT('Ctrl Pts',(9.53672456739186,0.35951284935727,4.5052776841562));
#8194=CARTESIAN_POINT('Ctrl Pts',(9.55308672779057,0.70168150119454,4.81072784092244));
#8195=CARTESIAN_POINT('Ctrl Pts',(9.56401498954576,0.786439952711774,5.10433647990876));
#8196=CARTESIAN_POINT('Ctrl Pts',(9.56947716492856,0.786459812675507,5.25186167987965));
#8197=CARTESIAN_POINT('Ctrl Pts',(6.53728986429481,0.791457584369433,5.24788844117082));
#8198=CARTESIAN_POINT('Ctrl Pts',(6.54278417054037,0.791437607580227,5.39628144910989));
#8199=CARTESIAN_POINT('Ctrl Pts',(6.55378249785739,0.706095273707095,5.69170633675433));
#8200=CARTESIAN_POINT('Ctrl Pts',(6.57024265516649,0.36194294842202,5.99886043512873));
#8201=CARTESIAN_POINT('Ctrl Pts',(6.58668071586564,-0.0921185468821841,
6.07520217151));
#8202=CARTESIAN_POINT('Ctrl Pts',(6.60308941390448,-0.516358086898658,5.8984073300043));
#8203=CARTESIAN_POINT('Ctrl Pts',(6.61947110658782,-0.781148791011006,5.52353693808151));
#8204=CARTESIAN_POINT('Ctrl Pts',(6.63582102071739,-0.805316342370628,5.06602826377862));
#8205=CARTESIAN_POINT('Ctrl Pts',(6.65214502140613,-0.582650139481846,4.66642310779825));
#8206=CARTESIAN_POINT('Ctrl Pts',(6.66571399431892,-0.248901893197726,4.48404923727362));
#8207=CARTESIAN_POINT('Ctrl Pts',(6.67656588894199,0.0453190981676558,4.46087101406537));
#8208=CARTESIAN_POINT('Ctrl Pts',(6.68467931966452,0.261934715600987,4.50488378698986));
#8209=CARTESIAN_POINT('Ctrl Pts',(6.69282445640136,0.457697749274946,4.60726786189105));
#8210=CARTESIAN_POINT('Ctrl Pts',(6.70086847028765,0.617302246342184,4.75966820326596));
#8211=CARTESIAN_POINT('Ctrl Pts',(6.70706046107289,0.700528406866124,4.90254788180947));
#8212=CARTESIAN_POINT('Ctrl Pts',(6.71094234002084,0.73818000698364,5.00497270204404));
#8213=CARTESIAN_POINT('Ctrl Pts',(6.71300604048302,0.753222836061835,5.05704788335984));
#8214=CARTESIAN_POINT('Ctrl Pts',(6.71539366913855,0.764820751174518,5.11043973498399));
#8215=CARTESIAN_POINT('Ctrl Pts',(6.71729493969799,0.77513823533657,5.18438795256581));
#8216=CARTESIAN_POINT('Ctrl Pts',(6.72080892065097,0.778397838898288,5.26987667291114));
#8217=CARTESIAN_POINT('Ctrl Pts',(6.73404917601244,0.763282472885072,5.4153514076569));
#8218=CARTESIAN_POINT('Ctrl Pts',(6.75227750605218,0.684423920730263,5.65860295458565));
#8219=CARTESIAN_POINT('Ctrl Pts',(6.77583192680458,0.483163536120546,5.8812916764581));
#8220=CARTESIAN_POINT('Ctrl Pts',(6.79769115526016,0.217124051184817,5.99794934103775));
#8221=CARTESIAN_POINT('Ctrl Pts',(6.8200508970381,-0.0700279426602678,6.03731900340549));
#8222=CARTESIAN_POINT('Ctrl Pts',(6.84761039460488,-0.426870037969381,5.93241072619413));
#8223=CARTESIAN_POINT('Ctrl Pts',(6.87950319278275,-0.70993595670243,5.61157204292273));
#8224=CARTESIAN_POINT('Ctrl Pts',(6.90997077663386,-0.788035834470172,5.21287382442806));
#8225=CARTESIAN_POINT('Ctrl Pts',(6.93913173491947,-0.671557590403463,4.84250449492373));
#8226=CARTESIAN_POINT('Ctrl Pts',(6.96815537921053,-0.393284210691007,4.57391816840494));
#8227=CARTESIAN_POINT('Ctrl Pts',(6.99706486303965,-0.0221876157039304,
4.47165816386748));
#8228=CARTESIAN_POINT('Ctrl Pts',(7.02584295552157,0.350991457602562,4.55877532096753));
#8229=CARTESIAN_POINT('Ctrl Pts',(7.05210448870892,0.612009659039021,4.79186963182615));
#8230=CARTESIAN_POINT('Ctrl Pts',(7.07588277971234,0.734898688262069,5.07852803586258));
#8231=CARTESIAN_POINT('Ctrl Pts',(7.10431766120651,0.748473408452173,5.45246510432511));
#8232=CARTESIAN_POINT('Ctrl Pts',(7.13495982630399,0.534772722166524,5.81756547683734));
#8233=CARTESIAN_POINT('Ctrl Pts',(7.16776257929051,0.13488149437605,5.99479462816283));
#8234=CARTESIAN_POINT('Ctrl Pts',(7.19574440030138,-0.236141062682786,5.96531940176238));
#8235=CARTESIAN_POINT('Ctrl Pts',(7.2177901342577,-0.482095505862949,5.8048713584837));
#8236=CARTESIAN_POINT('Ctrl Pts',(7.23397954190281,-0.609110618529052,5.63776724940332));
#8237=CARTESIAN_POINT('Ctrl Pts',(7.24783086290047,-0.689316230456583,5.47725973143276));
#8238=CARTESIAN_POINT('Ctrl Pts',(7.27200410720517,-0.748321146352422,5.16483188372505));
#8239=CARTESIAN_POINT('Ctrl Pts',(7.30634760775194,-0.573092566975053,4.72345680527967));
#8240=CARTESIAN_POINT('Ctrl Pts',(7.34725724358845,-0.061282166766824,4.47987864397431));
#8241=CARTESIAN_POINT('Ctrl Pts',(7.38786714614943,0.475093187126763,4.64821747196133));
#8242=CARTESIAN_POINT('Ctrl Pts',(7.4281808884662,0.752162744425484,5.13262048509692));
#8243=CARTESIAN_POINT('Ctrl Pts',(7.4682032841975,0.626465961329015,5.67275193455503));
#8244=CARTESIAN_POINT('Ctrl Pts',(7.50131695661259,0.246792245186754,5.92871444590393));
#8245=CARTESIAN_POINT('Ctrl Pts',(7.5276686028738,-0.0994340094365663,5.93948771421208));
#8246=CARTESIAN_POINT('Ctrl Pts',(7.54955183986769,-0.370434232319783,5.84438053773469));
#8247=CARTESIAN_POINT('Ctrl Pts',(7.57352589450599,-0.598389487794979,5.62068677638571));
#8248=CARTESIAN_POINT('Ctrl Pts',(7.59956122744709,-0.699716036243272,5.28908655646374));
#8249=CARTESIAN_POINT('Ctrl Pts',(7.62116131797656,-0.641707280988357,5.00738066570936));
#8250=CARTESIAN_POINT('Ctrl Pts',(7.63838529282816,-0.51956007976562,4.81959623297834));
#8251=CARTESIAN_POINT('Ctrl Pts',(7.65557203307511,-0.355360709732147,4.66755759217184));
#8252=CARTESIAN_POINT('Ctrl Pts',(7.67698583504015,-0.0901629384316624,
4.56431184492957));
#8253=CARTESIAN_POINT('Ctrl Pts',(7.7068428996256,0.305080740614273,4.61367696897994));
#8254=CARTESIAN_POINT('Ctrl Pts',(7.73442574632612,0.583537909728163,4.87373760666019));
#8255=CARTESIAN_POINT('Ctrl Pts',(7.75977754006825,0.667718615594098,5.19632076194103));
#8256=CARTESIAN_POINT('Ctrl Pts',(7.78505717843533,0.631510008529416,5.52614830373602));
#8257=CARTESIAN_POINT('Ctrl Pts',(7.81652540185333,0.359488412685916,5.86663423903951));
#8258=CARTESIAN_POINT('Ctrl Pts',(7.8509623942454,-0.11195737754036,5.93596459383563));
#8259=CARTESIAN_POINT('Ctrl Pts',(7.88213634505837,-0.477884403820245,5.73212312446919));
#8260=CARTESIAN_POINT('Ctrl Pts',(7.91009554163285,-0.659080145871757,5.40362312816743));
#8261=CARTESIAN_POINT('Ctrl Pts',(7.93099687270145,-0.642907181436071,5.12339682980178));
#8262=CARTESIAN_POINT('Ctrl Pts',(7.94490706513547,-0.571422723993177,4.95820274283118));
#8263=CARTESIAN_POINT('Ctrl Pts',(7.95185706711927,-0.524643983980393,4.8814350077215));
#8264=CARTESIAN_POINT('Ctrl Pts',(7.95880208822775,-0.467565899481637,4.81195386368381));
#8265=CARTESIAN_POINT('Ctrl Pts',(7.96959766060679,-0.364723690059826,4.71768110428399));
#8266=CARTESIAN_POINT('Ctrl Pts',(7.99039050550677,-0.123078463851595,4.58860653829953));
#8267=CARTESIAN_POINT('Ctrl Pts',(8.01804399168185,0.257517145674564,4.61775924801183));
#8268=CARTESIAN_POINT('Ctrl Pts',(8.04868561583974,0.564353076015046,4.89347251399917));
#8269=CARTESIAN_POINT('Ctrl Pts',(8.07620529241276,0.666448377061362,5.24794644083153));
#8270=CARTESIAN_POINT('Ctrl Pts',(8.10367692972224,0.564301163146253,5.60265220795495));
#8271=CARTESIAN_POINT('Ctrl Pts',(8.1311063371322,0.289652716430529,5.84793638333599));
#8272=CARTESIAN_POINT('Ctrl Pts',(8.15850125893085,-0.0729805081161587,
5.90966061766628));
#8273=CARTESIAN_POINT('Ctrl Pts',(8.18586870658201,-0.412536152354017,5.76911441682784));
#8274=CARTESIAN_POINT('Ctrl Pts',(8.2132161293016,-0.625176848653941,5.46974735708836));
#8275=CARTESIAN_POINT('Ctrl Pts',(8.24055084302331,-0.64600120604342,5.10329359763361));
#8276=CARTESIAN_POINT('Ctrl Pts',(8.26788027572269,-0.468758984456337,4.78196882475003));
#8277=CARTESIAN_POINT('Ctrl Pts',(8.29521182844757,-0.147733887802402,4.60412415342451));
#8278=CARTESIAN_POINT('Ctrl Pts',(8.32255291725131,0.218837928434283,4.62428040570159));
#8279=CARTESIAN_POINT('Ctrl Pts',(8.34991094871533,0.51871581464964,4.83645895467768));
#8280=CARTESIAN_POINT('Ctrl Pts',(8.37729320920923,0.659936333003741,5.17593146088852));
#8281=CARTESIAN_POINT('Ctrl Pts',(8.40470716926229,0.598866621643475,5.53894810421618));
#8282=CARTESIAN_POINT('Ctrl Pts',(8.43215968688036,0.353772456268368,5.81422753527536));
#8283=CARTESIAN_POINT('Ctrl Pts',(8.45965873301394,-0.00090935564745819,
5.91721890831774));
#8284=CARTESIAN_POINT('Ctrl Pts',(8.48261763222319,-0.297193347524019,5.832373515472));
#8285=CARTESIAN_POINT('Ctrl Pts',(8.5010170841175,-0.480578633759046,5.67772295629852));
#8286=CARTESIAN_POINT('Ctrl Pts',(8.51841470498558,-0.607165316349347,5.48959928016275));
#8287=CARTESIAN_POINT('Ctrl Pts',(8.53942561001488,-0.663406845956722,5.21544933331551));
#8288=CARTESIAN_POINT('Ctrl Pts',(8.5640860352834,-0.567257575299942,4.9015656424331));
#8289=CARTESIAN_POINT('Ctrl Pts',(8.5867469390981,-0.351851325775005,4.69008336352928));
#8290=CARTESIAN_POINT('Ctrl Pts',(8.60739743163042,-0.096086131236525,4.60049517355307));
#8291=CARTESIAN_POINT('Ctrl Pts',(8.63223189061381,0.230279583670253,4.6105197427705));
#8292=CARTESIAN_POINT('Ctrl Pts',(8.66337612152979,0.587448284147565,4.85122937163191));
#8293=CARTESIAN_POINT('Ctrl Pts',(8.70092976062667,0.705041399270903,5.35836385208443));
#8294=CARTESIAN_POINT('Ctrl Pts',(8.73867762820808,0.445619450565281,5.81178687736278));
#8295=CARTESIAN_POINT('Ctrl Pts',(8.77663330730281,-0.0561408892919382,
5.96913573334488));
#8296=CARTESIAN_POINT('Ctrl Pts',(8.808445476751,-0.453384395196325,5.77934323807869));
#8297=CARTESIAN_POINT('Ctrl Pts',(8.83401240846527,-0.631791197131727,5.49501245739173));
#8298=CARTESIAN_POINT('Ctrl Pts',(8.85965950209186,-0.697335209574664,5.16418731265143));
#8299=CARTESIAN_POINT('Ctrl Pts',(8.88757321050643,-0.558369116925368,4.80448896156448));
#8300=CARTESIAN_POINT('Ctrl Pts',(8.91780053797859,-0.220082182336464,4.58512097737996));
#8301=CARTESIAN_POINT('Ctrl Pts',(8.94382442090338,0.124888837012952,4.5574388084705));
#8302=CARTESIAN_POINT('Ctrl Pts',(8.97105550892288,0.456421745283963,4.7051036988583));
#8303=CARTESIAN_POINT('Ctrl Pts',(8.99951073066361,0.67902904616484,5.01548343676037));
#8304=CARTESIAN_POINT('Ctrl Pts',(9.02921638462349,0.703497102878303,5.41370372897262));
#8305=CARTESIAN_POINT('Ctrl Pts',(9.05908029308652,0.511342876044629,5.76565926471648));
#8306=CARTESIAN_POINT('Ctrl Pts',(9.08910308021335,0.159530985782651,5.96258159182352));
#8307=CARTESIAN_POINT('Ctrl Pts',(9.1192905439651,-0.245331677769252,5.94205029820737));
#8308=CARTESIAN_POINT('Ctrl Pts',(9.14963403851829,-0.579074368916519,5.70804769353886));
#8309=CARTESIAN_POINT('Ctrl Pts',(9.18015561858369,-0.738086143309763,5.33026750887227));
#8310=CARTESIAN_POINT('Ctrl Pts',(9.21080588468753,-0.671444952751785,4.92359816795805));
#8311=CARTESIAN_POINT('Ctrl Pts',(9.24169181514135,-0.39715715916767,4.61285379721767));
#8312=CARTESIAN_POINT('Ctrl Pts',(9.26741765382922,-0.0641141613479425,
4.51484111966771));
#8313=CARTESIAN_POINT('Ctrl Pts',(9.2883080329795,0.20420407129801,4.55162436548779));
#8314=CARTESIAN_POINT('Ctrl Pts',(9.30874254903957,0.452902156553228,4.66063468512768));
#8315=CARTESIAN_POINT('Ctrl Pts',(9.33077742980449,0.641269387174206,4.86904883099884));
#8316=CARTESIAN_POINT('Ctrl Pts',(9.34785549284168,0.715152744632072,5.0968004916225));
#8317=CARTESIAN_POINT('Ctrl Pts',(9.3602755301295,0.729323789248401,5.23347950840958));
#8318=CARTESIAN_POINT('Ctrl Pts',(9.36347417466056,0.726285408376634,5.31181320851451));
#8319=CARTESIAN_POINT('Ctrl Pts',(9.3652893660282,0.716598586410511,5.38174950648743));
#8320=CARTESIAN_POINT('Ctrl Pts',(9.36752488741168,0.705685048065471,5.43181944939317));
#8321=CARTESIAN_POINT('Ctrl Pts',(9.3694564647943,0.691630806425038,5.48052738798772));
#8322=CARTESIAN_POINT('Ctrl Pts',(9.37309440175116,0.656329841837037,5.57653790841529));
#8323=CARTESIAN_POINT('Ctrl Pts',(9.37890017016595,0.578305869960337,5.71051132408279));
#8324=CARTESIAN_POINT('Ctrl Pts',(9.38644471609761,0.428595584489612,5.85346785080748));
#8325=CARTESIAN_POINT('Ctrl Pts',(9.39408703335625,0.244909855550526,5.94954069523186));
#8326=CARTESIAN_POINT('Ctrl Pts',(9.40170234262852,0.0415804244967724,5.99086118264962));
#8327=CARTESIAN_POINT('Ctrl Pts',(9.41189201019065,-0.234704618905985,5.96909752603866));
#8328=CARTESIAN_POINT('Ctrl Pts',(9.42463859874445,-0.548259442305881,5.79780663399558));
#8329=CARTESIAN_POINT('Ctrl Pts',(9.43998582035194,-0.757710474392766,5.42204388560271));
#8330=CARTESIAN_POINT('Ctrl Pts',(9.4553698847925,-0.734901408935396,4.99163053542099));
#8331=CARTESIAN_POINT('Ctrl Pts',(9.47079546212505,-0.485807828284844,4.638295123357));
#8332=CARTESIAN_POINT('Ctrl Pts',(9.48626038209685,-0.0857752245725713,
4.47188596344179));
#8333=CARTESIAN_POINT('Ctrl Pts',(9.50176629783407,0.342505541926648,4.54371374658917));
#8334=CARTESIAN_POINT('Ctrl Pts',(9.51730779271675,0.667520614060755,4.83376258154226));
#8335=CARTESIAN_POINT('Ctrl Pts',(9.52769881073733,0.748180309761582,5.11286768976882));
#8336=CARTESIAN_POINT('Ctrl Pts',(9.53289545467617,0.748199204277581,5.25322128197838));
#8337=CARTESIAN_POINT('Ctrl Pts',(6.45999557459768,0.809254259106663,5.250752686764));
#8338=CARTESIAN_POINT('Ctrl Pts',(6.4656153380923,0.809233826166506,5.40253410767546));
#8339=CARTESIAN_POINT('Ctrl Pts',(6.47687026388547,0.721996890342757,5.70493974187684));
#8340=CARTESIAN_POINT('Ctrl Pts',(6.49375251888294,0.369096209330993,6.02010570850611));
#8341=CARTESIAN_POINT('Ctrl Pts',(6.51064436532253,-0.0975430423797339,
6.09868870265511));
#8342=CARTESIAN_POINT('Ctrl Pts',(6.52754122332568,-0.534494623907844,5.91673254754402));
#8343=CARTESIAN_POINT('Ctrl Pts',(6.54444265909054,-0.80783698079355,5.52997825893372));
#8344=CARTESIAN_POINT('Ctrl Pts',(6.56134181204163,-0.832953247332849,5.05695964598303));
#8345=CARTESIAN_POINT('Ctrl Pts',(6.57824957990225,-0.602395099269935,4.64291194589478));
#8346=CARTESIAN_POINT('Ctrl Pts',(6.59232904971087,-0.256033804084603,4.45351553617427));
#8347=CARTESIAN_POINT('Ctrl Pts',(6.60360883315493,0.0498248485384295,4.42939603265042));
#8348=CARTESIAN_POINT('Ctrl Pts',(6.61205006886682,0.275217590098315,4.47517626334091));
#8349=CARTESIAN_POINT('Ctrl Pts',(6.62053196867004,0.479123848697043,4.58179723556108));
#8350=CARTESIAN_POINT('Ctrl Pts',(6.62891789718303,0.645505596832454,4.74066879125782));
#8351=CARTESIAN_POINT('Ctrl Pts',(6.63537635713297,0.732382034014202,4.88975766855534));
#8352=CARTESIAN_POINT('Ctrl Pts',(6.63943352928247,0.771687074389179,4.99674959091469));
#8353=CARTESIAN_POINT('Ctrl Pts',(6.64159806006668,0.787546974765718,5.05148060438962));
#8354=CARTESIAN_POINT('Ctrl Pts',(6.64410012271561,0.799529214601232,5.10718632608853));
#8355=CARTESIAN_POINT('Ctrl Pts',(6.64598144448542,0.810256089987908,5.18246997920793));
#8356=CARTESIAN_POINT('Ctrl Pts',(6.64995259301237,0.813716246088648,5.27746723531887));
#8357=CARTESIAN_POINT('Ctrl Pts',(6.66376398254105,0.797925459082292,5.42854929342793));
#8358=CARTESIAN_POINT('Ctrl Pts',(6.68284421486437,0.715379131781609,5.68363809114948));
#8359=CARTESIAN_POINT('Ctrl Pts',(6.70758451472148,0.504157330037584,5.9173892723336));
#8360=CARTESIAN_POINT('Ctrl Pts',(6.73061771554503,0.223813352606992,6.04046536159552));
#8361=CARTESIAN_POINT('Ctrl Pts',(6.75422019989529,-0.0793026005240917,
6.08203779050005));
#8362=CARTESIAN_POINT('Ctrl Pts',(6.783391300017,-0.457122076023753,5.97122820611254));
#8363=CARTESIAN_POINT('Ctrl Pts',(6.81727322163079,-0.758063258382887,5.63048355896042));
#8364=CARTESIAN_POINT('Ctrl Pts',(6.84975212437726,-0.84150197430614,5.20546023039942));
#8365=CARTESIAN_POINT('Ctrl Pts',(6.88093505637388,-0.717082698284182,4.80931695387591));
#8366=CARTESIAN_POINT('Ctrl Pts',(6.91206488791777,-0.418682655365162,4.52109212196899));
#8367=CARTESIAN_POINT('Ctrl Pts',(6.94316889035763,-0.0194331785847506,
4.41091747648985));
#8368=CARTESIAN_POINT('Ctrl Pts',(6.97422006674403,0.383283395774545,4.5047807265211));
#8369=CARTESIAN_POINT('Ctrl Pts',(7.00263321675371,0.665816074281837,4.75690914542035));
#8370=CARTESIAN_POINT('Ctrl Pts',(7.02842338889131,0.799161055122401,5.06782415611563));
#8371=CARTESIAN_POINT('Ctrl Pts',(7.05932459014209,0.814003215770462,5.47420123361874));
#8372=CARTESIAN_POINT('Ctrl Pts',(7.09271704357918,0.581339250156787,5.87227691308354));
#8373=CARTESIAN_POINT('Ctrl Pts',(7.12857742875714,0.144206008983758,6.0661807345317));
#8374=CARTESIAN_POINT('Ctrl Pts',(7.15923642529593,-0.262355703606541,6.03398209938642));
#8375=CARTESIAN_POINT('Ctrl Pts',(7.18344185505573,-0.532486116512524,5.85786320372732));
#8376=CARTESIAN_POINT('Ctrl Pts',(7.2012453498512,-0.672177603901523,5.67409256107297));
#8377=CARTESIAN_POINT('Ctrl Pts',(7.21648898591514,-0.760453017446425,5.49744398399632));
#8378=CARTESIAN_POINT('Ctrl Pts',(7.24312182063594,-0.825515825922649,5.15323254742201));
#8379=CARTESIAN_POINT('Ctrl Pts',(7.28103894373652,-0.632275153963754,4.665803037915));
#8380=CARTESIAN_POINT('Ctrl Pts',(7.3263220317354,-0.0658377557766746,4.39591133185141));
#8381=CARTESIAN_POINT('Ctrl Pts',(7.37137511216033,0.52933208569028,4.58245170719848));
#8382=CARTESIAN_POINT('Ctrl Pts',(7.41618714911392,0.837507063114166,5.12082756912408));
#8383=CARTESIAN_POINT('Ctrl Pts',(7.46074788044844,0.697712679683577,5.7222691996181));
#8384=CARTESIAN_POINT('Ctrl Pts',(7.49766411510097,0.274482978524602,6.00771346693692));
#8385=CARTESIAN_POINT('Ctrl Pts',(7.52706281789054,-0.111787067247916,6.01974462374398));
#8386=CARTESIAN_POINT('Ctrl Pts',(7.55148599389226,-0.414241243525464,5.9136075100233));
#8387=CARTESIAN_POINT('Ctrl Pts',(7.57825173171333,-0.668747225075187,5.66387265100419));
#8388=CARTESIAN_POINT('Ctrl Pts',(7.60732576554949,-0.781899451692313,5.29357550966227));
#8389=CARTESIAN_POINT('Ctrl Pts',(7.63144825543078,-0.717112820017105,4.97897772631035));
#8390=CARTESIAN_POINT('Ctrl Pts',(7.65068202749864,-0.580711872249469,4.76928606869434));
#8391=CARTESIAN_POINT('Ctrl Pts',(7.66987254015019,-0.397368841933043,4.59952785513379));
#8392=CARTESIAN_POINT('Ctrl Pts',(7.6937789668775,-0.101308809637811,4.48428345691279));
#8393=CARTESIAN_POINT('Ctrl Pts',(7.72709483698664,0.339719003758443,4.53940207795531));
#8394=CARTESIAN_POINT('Ctrl Pts',(7.75785104299278,0.650135480752808,4.82942921168495));
#8395=CARTESIAN_POINT('Ctrl Pts',(7.78609058120298,0.743868677952219,5.18874820762418));
#8396=CARTESIAN_POINT('Ctrl Pts',(7.81422927914199,0.703540142915436,5.5558670520897));
#8397=CARTESIAN_POINT('Ctrl Pts',(7.84921332159718,0.401011003875481,5.93425427218728));
#8398=CARTESIAN_POINT('Ctrl Pts',(7.88741640054593,-0.121987511272621,6.01093434276299));
#8399=CARTESIAN_POINT('Ctrl Pts',(7.92192473853693,-0.526942532140401,5.78518530972292));
#8400=CARTESIAN_POINT('Ctrl Pts',(7.95281213238897,-0.726978532166836,5.42226623438594));
#8401=CARTESIAN_POINT('Ctrl Pts',(7.97585068557117,-0.709046349578469,5.11344268985378));
#8402=CARTESIAN_POINT('Ctrl Pts',(7.99115589437824,-0.630392934079408,4.93169356901783));
#8403=CARTESIAN_POINT('Ctrl Pts',(7.99879796520076,-0.57895613111009,4.84728516828961));
#8404=CARTESIAN_POINT('Ctrl Pts',(8.00642950767667,-0.516235309566051,4.77094091026953));
#8405=CARTESIAN_POINT('Ctrl Pts',(8.01828457552326,-0.403306159141596,4.66742318077098));
#8406=CARTESIAN_POINT('Ctrl Pts',(8.04109084512299,-0.138232407133623,4.52591534703238));
#8407=CARTESIAN_POINT('Ctrl Pts',(8.07133153658797,0.277933340832045,4.55808290998239));
#8408=CARTESIAN_POINT('Ctrl Pts',(8.10472163981035,0.612088745400635,4.85866032793836));
#8409=CARTESIAN_POINT('Ctrl Pts',(8.13461238013838,0.722784116446006,5.24364859132425));
#8410=CARTESIAN_POINT('Ctrl Pts',(8.16434352076723,0.612051583526427,5.62741670623071));
#8411=CARTESIAN_POINT('Ctrl Pts',(8.19391894017278,0.315829296131672,5.89168368886382));
#8412=CARTESIAN_POINT('Ctrl Pts',(8.22334148667717,-0.073615600048539,5.95774627858268));
#8413=CARTESIAN_POINT('Ctrl Pts',(8.2526148686265,-0.436664486169176,5.80722357120211));
#8414=CARTESIAN_POINT('Ctrl Pts',(8.2817428109828,-0.662913169596188,5.48828297433822));
#8415=CARTESIAN_POINT('Ctrl Pts',(8.31072941188433,-0.684744084908157,5.09973973531902));
#8416=CARTESIAN_POINT('Ctrl Pts',(8.33957899299675,-0.497454685626346,4.76072710518954));
#8417=CARTESIAN_POINT('Ctrl Pts',(8.36829613554204,-0.160092402883954,4.57412892458932));
#8418=CARTESIAN_POINT('Ctrl Pts',(8.39688569797962,0.223129005271864,4.59546606782747));
#8419=CARTESIAN_POINT('Ctrl Pts',(8.42535271673465,0.53494485713908,4.81642132873474));
#8420=CARTESIAN_POINT('Ctrl Pts',(8.4537025819109,0.68087147706904,5.16792102261738));
#8421=CARTESIAN_POINT('Ctrl Pts',(8.48194066992712,0.617705346936381,5.54172542134465));
#8422=CARTESIAN_POINT('Ctrl Pts',(8.51007311419913,0.366388819790279,5.82356941025869));
#8423=CARTESIAN_POINT('Ctrl Pts',(8.53810505214009,0.00483044772678114,
5.92826112657717));
#8424=CARTESIAN_POINT('Ctrl Pts',(8.56138803027302,-0.295480207153548,5.84201972788554));
#8425=CARTESIAN_POINT('Ctrl Pts',(8.57996830905769,-0.480604419515746,5.68583764688899));
#8426=CARTESIAN_POINT('Ctrl Pts',(8.59748940753691,-0.608047312296436,5.4963666433294));
#8427=CARTESIAN_POINT('Ctrl Pts',(8.61857918989552,-0.664302447321313,5.221247595173));
#8428=CARTESIAN_POINT('Ctrl Pts',(8.64320525787944,-0.56811782681272,4.90788926095751));
#8429=CARTESIAN_POINT('Ctrl Pts',(8.66573081669197,-0.353908674160115,4.69784543743962));
#8430=CARTESIAN_POINT('Ctrl Pts',(8.6861712326096,-0.100775202667368,4.60925906979357));
#8431=CARTESIAN_POINT('Ctrl Pts',(8.71066377776687,0.221098389390166,4.61926760882404));
#8432=CARTESIAN_POINT('Ctrl Pts',(8.74122227864302,0.571184388107263,4.85585622113353));
#8433=CARTESIAN_POINT('Ctrl Pts',(8.7778130831244,0.685078508551102,5.3500353521348));
#8434=CARTESIAN_POINT('Ctrl Pts',(8.81434182728614,0.433536012261789,5.78839143480342));
#8435=CARTESIAN_POINT('Ctrl Pts',(8.85082537278578,-0.0488556501951366,
5.93899861839975));
#8436=CARTESIAN_POINT('Ctrl Pts',(8.88120666328966,-0.427908344867109,5.75733976610283));
#8437=CARTESIAN_POINT('Ctrl Pts',(8.90550515735323,-0.597345302500117,5.48714044975464));
#8438=CARTESIAN_POINT('Ctrl Pts',(8.92980208102577,-0.65933912822784,5.1737060918429));
#8439=CARTESIAN_POINT('Ctrl Pts',(8.95613036104259,-0.527930599875553,4.83463896743551));
#8440=CARTESIAN_POINT('Ctrl Pts',(8.98449755789417,-0.210401683525278,4.62895776604595));
#8441=CARTESIAN_POINT('Ctrl Pts',(9.0088288410772,0.112116097503262,4.60321902465812));
#8442=CARTESIAN_POINT('Ctrl Pts',(9.03419634827837,0.420871346111283,4.74090449262632));
#8443=CARTESIAN_POINT('Ctrl Pts',(9.06061136980048,0.627320838871634,5.02907173541959));
#8444=CARTESIAN_POINT('Ctrl Pts',(9.0880818259389,0.649761518074933,5.39726951746239));
#8445=CARTESIAN_POINT('Ctrl Pts',(9.11560011871394,0.472584972123624,5.72143515200543));
#8446=CARTESIAN_POINT('Ctrl Pts',(9.14317100932603,0.149484864062567,5.90209915790658));
#8447=CARTESIAN_POINT('Ctrl Pts',(9.17080492383359,-0.221056026697281,5.88315245478754));
#8448=CARTESIAN_POINT('Ctrl Pts',(9.19849913151102,-0.525520480330484,5.66949773032316));
#8449=CARTESIAN_POINT('Ctrl Pts',(9.22627859524352,-0.670094333871429,5.32565914727594));
#8450=CARTESIAN_POINT('Ctrl Pts',(9.25410461778296,-0.609472890704072,4.95654943349016));
#8451=CARTESIAN_POINT('Ctrl Pts',(9.28207813619629,-0.360990719160832,4.67522249318265));
#8452=CARTESIAN_POINT('Ctrl Pts',(9.30533083985056,-0.0599919750808904,
4.58674525641782));
#8453=CARTESIAN_POINT('Ctrl Pts',(9.32418289262162,0.18212513724471,4.619946808137));
#8454=CARTESIAN_POINT('Ctrl Pts',(9.34260730899467,0.406349206044995,4.71826942359272));
#8455=CARTESIAN_POINT('Ctrl Pts',(9.36245403617579,0.575921431786298,4.90591614259015));
#8456=CARTESIAN_POINT('Ctrl Pts',(9.377810035467,0.642356264883323,5.11081796432513));
#8457=CARTESIAN_POINT('Ctrl Pts',(9.38896656846135,0.655091434360625,5.23342471494882));
#8458=CARTESIAN_POINT('Ctrl Pts',(9.39191714275027,0.652347070971567,5.3052545908254));
#8459=CARTESIAN_POINT('Ctrl Pts',(9.3935201178333,0.643661393979997,5.36754984112474));
#8460=CARTESIAN_POINT('Ctrl Pts',(9.39552997481224,0.63389436064975,5.41250038978432));
#8461=CARTESIAN_POINT('Ctrl Pts',(9.39726703478231,0.621234849848933,5.45632929190797));
#8462=CARTESIAN_POINT('Ctrl Pts',(9.40053483057608,0.589538443172086,5.54255337995261));
#8463=CARTESIAN_POINT('Ctrl Pts',(9.40574774560895,0.51947566576292,5.66283951997694));
#8464=CARTESIAN_POINT('Ctrl Pts',(9.41252022585287,0.385101609192844,5.79115143286413));
#8465=CARTESIAN_POINT('Ctrl Pts',(9.41937850660532,0.220268888907917,5.87736017606902));
#8466=CARTESIAN_POINT('Ctrl Pts',(9.42621082062533,0.0378591974212147,5.91442689341244));
#8467=CARTESIAN_POINT('Ctrl Pts',(9.43535036503967,-0.209940808359547,5.89490298832899));
#8468=CARTESIAN_POINT('Ctrl Pts',(9.44678065086537,-0.491072382960274,5.74130501383786));
#8469=CARTESIAN_POINT('Ctrl Pts',(9.46053662841775,-0.678774393287174,5.40451551930697));
#8470=CARTESIAN_POINT('Ctrl Pts',(9.47432096030564,-0.658324053358711,5.01889497646438));
#8471=CARTESIAN_POINT('Ctrl Pts',(9.48813807913884,-0.435204188314633,4.70241739537075));
#8472=CARTESIAN_POINT('Ctrl Pts',(9.50198713723629,-0.0769945315313026,
4.55342872186793));
#8473=CARTESIAN_POINT('Ctrl Pts',(9.51586821916381,0.30642949046769,4.61770812146408));
#8474=CARTESIAN_POINT('Ctrl Pts',(9.52978247204756,0.597360200833237,4.87739913147432));
#8475=CARTESIAN_POINT('Ctrl Pts',(9.53907878780185,0.669558525647519,5.127085468639));
#8476=CARTESIAN_POINT('Ctrl Pts',(9.54373454600902,0.669575453553099,5.25283054498549));
#8477=CARTESIAN_POINT('Ctrl Pts',(6.3975642485275,0.760068228697932,5.2530576083404));
#8478=CARTESIAN_POINT('Ctrl Pts',(6.40284604135377,0.760049024587858,5.39571094613652));
#8479=CARTESIAN_POINT('Ctrl Pts',(6.41342366827503,0.678086500584757,5.67989070809738));
#8480=CARTESIAN_POINT('Ctrl Pts',(6.42932406057163,0.345838155681425,5.97679828638407));
#8481=CARTESIAN_POINT('Ctrl Pts',(6.44525966089941,-0.0943537342223277,
6.05101384381127));
#8482=CARTESIAN_POINT('Ctrl Pts',(6.46122925955391,-0.507332803137623,5.87917628308332));
#8483=CARTESIAN_POINT('Ctrl Pts',(6.47723247686921,-0.766215951571805,5.5130774349882));
#8484=CARTESIAN_POINT('Ctrl Pts',(6.4932655429891,-0.790163937030003,5.06441564556022));
#8485=CARTESIAN_POINT('Ctrl Pts',(6.50933478250395,-0.571182355221987,4.67090374066804));
#8486=CARTESIAN_POINT('Ctrl Pts',(6.52274298444712,-0.241477409664008,4.49049679612232));
#8487=CARTESIAN_POINT('Ctrl Pts',(6.53349756884893,0.0501147882500171,4.46748118948392));
#8488=CARTESIAN_POINT('Ctrl Pts',(6.54155389312568,0.265195219859689,4.51115221205005));
#8489=CARTESIAN_POINT('Ctrl Pts',(6.54965647563047,0.459973714137355,4.6129814833824));
#8490=CARTESIAN_POINT('Ctrl Pts',(6.5576758012139,0.619037348482741,4.76486078836297));
#8491=CARTESIAN_POINT('Ctrl Pts',(6.5638565028091,0.702214918141095,4.90753456196431));
#8492=CARTESIAN_POINT('Ctrl Pts',(6.56774522291797,0.739840261363108,5.01001808408939));
#8493=CARTESIAN_POINT('Ctrl Pts',(6.56982725311109,0.755173986750213,5.06276611003264));
#8494=CARTESIAN_POINT('Ctrl Pts',(6.57223182121529,0.766523132772943,5.11606099522602));
#8495=CARTESIAN_POINT('Ctrl Pts',(6.57393262316656,0.776748482011025,5.18626717050706));
#8496=CARTESIAN_POINT('Ctrl Pts',(6.57802798038273,0.780117929748685,5.28278909253043));
#8497=CARTESIAN_POINT('Ctrl Pts',(6.59124494998433,0.764983429094594,5.42671920642507));
#8498=CARTESIAN_POINT('Ctrl Pts',(6.60956554315219,0.68572326715126,5.67210008102203));
#8499=CARTESIAN_POINT('Ctrl Pts',(6.63342570307357,0.482275698626895,5.89729441612607));
#8500=CARTESIAN_POINT('Ctrl Pts',(6.65569976703258,0.211186373881766,6.01644845156957));
#8501=CARTESIAN_POINT('Ctrl Pts',(6.67857023173211,-0.0824821450646381,
6.05674685227899));
#8502=CARTESIAN_POINT('Ctrl Pts',(6.70693191311676,-0.449782403728053,5.94930974724307));
#8503=CARTESIAN_POINT('Ctrl Pts',(6.74000644362055,-0.743697403464958,5.61692476045587));
#8504=CARTESIAN_POINT('Ctrl Pts',(6.77183780370126,-0.825660357870783,5.20051970189362));
#8505=CARTESIAN_POINT('Ctrl Pts',(6.80251278275663,-0.703475060709293,4.81085211691783));
#8506=CARTESIAN_POINT('Ctrl Pts',(6.83325307834601,-0.409020216329708,4.52616875178095));
#8507=CARTESIAN_POINT('Ctrl Pts',(6.86407778139747,-0.013438207806227,4.41681026053004));
#8508=CARTESIAN_POINT('Ctrl Pts',(6.89496847918126,0.387190546300914,4.50998959025875));
#8509=CARTESIAN_POINT('Ctrl Pts',(6.92334526410876,0.669439165256199,4.76162282320026));
#8510=CARTESIAN_POINT('Ctrl Pts',(6.94918439495235,0.803100128876369,5.07308158460193));
#8511=CARTESIAN_POINT('Ctrl Pts',(6.98023347108384,0.818138478146011,5.48132682598222));
#8512=CARTESIAN_POINT('Ctrl Pts',(7.01393507577349,0.583765048880111,5.88323952969222));
#8513=CARTESIAN_POINT('Ctrl Pts',(7.05029034196779,0.140714106057853,6.08003730568266));
#8514=CARTESIAN_POINT('Ctrl Pts',(7.08149210594045,-0.273016084884725,6.04746437682534));
#8515=CARTESIAN_POINT('Ctrl Pts',(7.10622343068897,-0.549029305695015,5.86769627218021));
#8516=CARTESIAN_POINT('Ctrl Pts',(7.1244552483263,-0.692090135230285,5.67952629490147));
#8517=CARTESIAN_POINT('Ctrl Pts',(7.14008798549728,-0.782618105115043,5.49838936905692));
#8518=CARTESIAN_POINT('Ctrl Pts',(7.16745761696029,-0.849577897570751,5.14473853593693));
#8519=CARTESIAN_POINT('Ctrl Pts',(7.20658941040099,-0.650684341966546,4.64158371398262));
#8520=CARTESIAN_POINT('Ctrl Pts',(7.25357695572029,-0.0633045461604468,
4.3609623615544));
#8521=CARTESIAN_POINT('Ctrl Pts',(7.30057733164244,0.557708033944997,4.55491612196963));
#8522=CARTESIAN_POINT('Ctrl Pts',(7.34757286249331,0.881406337177324,5.11912513726633));
#8523=CARTESIAN_POINT('Ctrl Pts',(7.39454538146955,0.734686256930202,5.75319528327261));
#8524=CARTESIAN_POINT('Ctrl Pts',(7.43365687136522,0.286617000227074,6.05598265751437));
#8525=CARTESIAN_POINT('Ctrl Pts',(7.46491538644837,-0.124078879570498,6.06888030729612));
#8526=CARTESIAN_POINT('Ctrl Pts',(7.49094515362771,-0.446422101358953,5.95583388766042));
#8527=CARTESIAN_POINT('Ctrl Pts',(7.51955536822179,-0.718525845560669,5.68904753107812));
#8528=CARTESIAN_POINT('Ctrl Pts',(7.55072731520184,-0.839977697613594,5.29213009146162));
#8529=CARTESIAN_POINT('Ctrl Pts',(7.57666686463738,-0.770445104836072,4.95383991243434));
#8530=CARTESIAN_POINT('Ctrl Pts',(7.59739316080166,-0.623484139109556,4.7278712732606));
#8531=CARTESIAN_POINT('Ctrl Pts',(7.61810309328136,-0.425660210814252,4.54466649182984));
#8532=CARTESIAN_POINT('Ctrl Pts',(7.64396055049064,-0.105529779735548,4.4199311002941));
#8533=CARTESIAN_POINT('Ctrl Pts',(7.68008681845853,0.372701727578117,4.47952100368038));
#8534=CARTESIAN_POINT('Ctrl Pts',(7.71355248212602,0.710651761559828,4.79483205441596));
#8535=CARTESIAN_POINT('Ctrl Pts',(7.7443629084714,0.812996711285813,5.18686102863723));
#8536=CARTESIAN_POINT('Ctrl Pts',(7.77512035944637,0.768988465478849,5.58810403940493));
#8537=CARTESIAN_POINT('Ctrl Pts',(7.81346225286718,0.437720151424322,6.00298785716469));
#8538=CARTESIAN_POINT('Ctrl Pts',(7.85546711372016,-0.137253206275788,6.08763408005374));
#8539=CARTESIAN_POINT('Ctrl Pts',(7.89350847994605,-0.583738633090295,5.83892102537973));
#8540=CARTESIAN_POINT('Ctrl Pts',(7.92763049904828,-0.804821403375952,5.43809078417017));
#8541=CARTESIAN_POINT('Ctrl Pts',(7.9531308415908,-0.785069701277599,5.09628801507745));
#8542=CARTESIAN_POINT('Ctrl Pts',(7.97008865655783,-0.697928181014753,4.89491411877532));
#8543=CARTESIAN_POINT('Ctrl Pts',(7.97855948171228,-0.640915735564249,4.80135284223213));
#8544=CARTESIAN_POINT('Ctrl Pts',(7.98702215880035,-0.571366863372613,4.71669331991059));
#8545=CARTESIAN_POINT('Ctrl Pts',(8.00017374436506,-0.446089544766635,4.60185560278705));
#8546=CARTESIAN_POINT('Ctrl Pts',(8.02549283150456,-0.151845066061863,4.44472298246148));
#8547=CARTESIAN_POINT('Ctrl Pts',(8.05911401414102,0.310851653233882,4.4803431473172));
#8548=CARTESIAN_POINT('Ctrl Pts',(8.09628982312233,0.682960272889444,4.81493413878844));
#8549=CARTESIAN_POINT('Ctrl Pts',(8.12960374965605,0.806389045514395,5.24399675485307));
#8550=CARTESIAN_POINT('Ctrl Pts',(8.16276733565534,0.682922920155554,5.67208701553495));
#8551=CARTESIAN_POINT('Ctrl Pts',(8.19577818693008,0.352311944327571,5.9670837080692));
#8552=CARTESIAN_POINT('Ctrl Pts',(8.22863264240994,-0.0825629153572059,
6.04087783376966));
#8553=CARTESIAN_POINT('Ctrl Pts',(8.26132800369485,-0.488067210769859,5.87276577273915));
#8554=CARTESIAN_POINT('Ctrl Pts',(8.29386155280421,-0.74077637673532,5.51652145653297));
#8555=CARTESIAN_POINT('Ctrl Pts',(8.3262310099455,-0.765141573786744,5.08261410411509));
#8556=CARTESIAN_POINT('Ctrl Pts',(8.35843433417891,-0.556044846512561,4.70418551870374));
#8557=CARTESIAN_POINT('Ctrl Pts',(8.39046982367808,-0.179657347321662,4.49604889689588));
#8558=CARTESIAN_POINT('Ctrl Pts',(8.42233607195163,0.247511742503061,4.5198871077102));
#8559=CARTESIAN_POINT('Ctrl Pts',(8.45403200084779,0.594683503231845,4.76597769364031));
#8560=CARTESIAN_POINT('Ctrl Pts',(8.48555684223994,0.756894001188261,5.15690766378376));
#8561=CARTESIAN_POINT('Ctrl Pts',(8.51691015446463,0.68666220127433,5.57197297916182));
#8562=CARTESIAN_POINT('Ctrl Pts',(8.54809180995931,0.407998968484439,5.88433263611551));
#8563=CARTESIAN_POINT('Ctrl Pts',(8.57910201533282,0.00795162764025913,
6.00004580282724));
#8564=CARTESIAN_POINT('Ctrl Pts',(8.6048013940002,-0.323544528379635,5.90474031577638));
#8565=CARTESIAN_POINT('Ctrl Pts',(8.62527588995087,-0.527538523543061,5.73261036130886));
#8566=CARTESIAN_POINT('Ctrl Pts',(8.64455963194646,-0.667794018511264,5.52405322458113));
#8567=CARTESIAN_POINT('Ctrl Pts',(8.66772398150025,-0.729516788746334,5.22178980165561));
#8568=CARTESIAN_POINT('Ctrl Pts',(8.6947115213019,-0.623992833684527,4.87839995894372));
#8569=CARTESIAN_POINT('Ctrl Pts',(8.71932941129584,-0.389778889903979,4.64889155370676));
#8570=CARTESIAN_POINT('Ctrl Pts',(8.74161491094236,-0.113760951060223,4.55235377325117));
#8571=CARTESIAN_POINT('Ctrl Pts',(8.76826131811639,0.236463642093971,4.56332162481603));
#8572=CARTESIAN_POINT('Ctrl Pts',(8.8013895184305,0.615841184389589,4.82017769980994));
#8573=CARTESIAN_POINT('Ctrl Pts',(8.84086340331569,0.738210427752782,5.35350219278022));
#8574=CARTESIAN_POINT('Ctrl Pts',(8.88006472675475,0.46774700707792,5.82374541850904));
#8575=CARTESIAN_POINT('Ctrl Pts',(8.9190021131565,-0.0473547807328733,5.9839561652154));
#8576=CARTESIAN_POINT('Ctrl Pts',(8.95123692710172,-0.449393545951968,5.79074568682316));
#8577=CARTESIAN_POINT('Ctrl Pts',(8.97690325278144,-0.628299851082753,5.50527526375753));
#8578=CARTESIAN_POINT('Ctrl Pts',(9.00249067541009,-0.69348799230158,5.17511262738361));
#8579=CARTESIAN_POINT('Ctrl Pts',(9.0300818610813,-0.555353587350565,4.81986222419062));
#8580=CARTESIAN_POINT('Ctrl Pts',(9.0596537824972,-0.224198845203747,4.60565111673752));
#8581=CARTESIAN_POINT('Ctrl Pts',(9.08490549546368,0.110568591021175,4.57910492629159));
#8582=CARTESIAN_POINT('Ctrl Pts',(9.11111456267047,0.429517962801524,4.72156968021327));
#8583=CARTESIAN_POINT('Ctrl Pts',(9.13826748581402,0.641572051369251,5.01801495571582));
#8584=CARTESIAN_POINT('Ctrl Pts',(9.16636064343759,0.664243389357046,5.39466135553552));
#8585=CARTESIAN_POINT('Ctrl Pts',(9.19435473755382,0.483712991221918,5.72436734483168));
#8586=CARTESIAN_POINT('Ctrl Pts',(9.22225428967748,0.156556617497767,5.90697725081521));
#8587=CARTESIAN_POINT('Ctrl Pts',(9.25006860981886,-0.216462968184482,5.88762228369914));
#8588=CARTESIAN_POINT('Ctrl Pts',(9.27779490424495,-0.521173298004424,5.67345613827036));
#8589=CARTESIAN_POINT('Ctrl Pts',(9.30545764377868,-0.664905802214252,5.33089556329931));
#8590=CARTESIAN_POINT('Ctrl Pts',(9.33301923890341,-0.604574180753094,4.96529698499221));
#8591=CARTESIAN_POINT('Ctrl Pts',(9.36057937654899,-0.359512498236151,4.68826678446829));
#8592=CARTESIAN_POINT('Ctrl Pts',(9.38336763883071,-0.0644150007369484,
4.60181005320466));
#8593=CARTESIAN_POINT('Ctrl Pts',(9.40177229277858,0.171957864695282,4.63424204726826));
#8594=CARTESIAN_POINT('Ctrl Pts',(9.41971547820392,0.390339392509962,4.73014944693566));
#8595=CARTESIAN_POINT('Ctrl Pts',(9.43896126596102,0.554595856232393,4.91197438114008));
#8596=CARTESIAN_POINT('Ctrl Pts',(9.45378482555719,0.618730996160634,5.11023167780338));
#8597=CARTESIAN_POINT('Ctrl Pts',(9.46450812670568,0.630993754219246,5.22742155461715));
#8598=CARTESIAN_POINT('Ctrl Pts',(9.46764503127636,0.628297080576472,5.30219028275335));
#8599=CARTESIAN_POINT('Ctrl Pts',(9.46908405130908,0.619988284606207,5.36019955318967));
#8600=CARTESIAN_POINT('Ctrl Pts',(9.47102628349308,0.610719630094374,5.40339518180637));
#8601=CARTESIAN_POINT('Ctrl Pts',(9.47270676110673,0.598391365633221,5.44590610393438));
#8602=CARTESIAN_POINT('Ctrl Pts',(9.47585389932824,0.567911563922736,5.52888863921652));
#8603=CARTESIAN_POINT('Ctrl Pts',(9.48086157752316,0.500540513684368,5.6444944560202));
#8604=CARTESIAN_POINT('Ctrl Pts',(9.4873632826241,0.371548176565824,5.76766631765112));
#8605=CARTESIAN_POINT('Ctrl Pts',(9.49393826309572,0.213479131284237,5.85031521547837));
#8606=CARTESIAN_POINT('Ctrl Pts',(9.5004811182654,0.0387777611901389,5.88579913080903));
#8607=CARTESIAN_POINT('Ctrl Pts',(9.50922333920638,-0.198282351728511,5.86709693896304));
#8608=CARTESIAN_POINT('Ctrl Pts',(9.52013452774334,-0.46667830079645,5.72032868888011));
#8609=CARTESIAN_POINT('Ctrl Pts',(9.53323680753399,-0.645398555208325,5.39939701305271));
#8610=CARTESIAN_POINT('Ctrl Pts',(9.54633608057676,-0.625836293082998,5.03285670636973));
#8611=CARTESIAN_POINT('Ctrl Pts',(9.55943542919992,-0.414150298918583,4.73277350781654));
#8612=CARTESIAN_POINT('Ctrl Pts',(9.57253867700424,-0.0751472013293622,
4.59190807185631));
#8613=CARTESIAN_POINT('Ctrl Pts',(9.58564225817841,0.286850803022957,4.65267462198366));
#8614=CARTESIAN_POINT('Ctrl Pts',(9.59875166752506,0.560859734073248,4.89747222799095));
#8615=CARTESIAN_POINT('Ctrl Pts',(9.6074850747912,0.628637838448434,5.13210373452291));
#8616=CARTESIAN_POINT('Ctrl Pts',(9.61186183958885,0.628653751959821,5.25031361552224));
#8617=CARTESIAN_POINT('Ctrl Pts',(6.39751711228746,0.680624720495572,5.25304865882655));
#8618=CARTESIAN_POINT('Ctrl Pts',(6.40225233315809,0.680607503670563,5.38093990420756));
#8619=CARTESIAN_POINT('Ctrl Pts',(6.41172205109112,0.607201745611839,5.63535890108503));
#8620=CARTESIAN_POINT('Ctrl Pts',(6.4259709706028,0.309516653578047,5.90146181902454));
#8621=CARTESIAN_POINT('Ctrl Pts',(6.44025312148205,-0.0850383123659948,
5.96797084256395));
#8622=CARTESIAN_POINT('Ctrl Pts',(6.45457324150139,-0.455365964413035,5.81391716320603));
#8623=CARTESIAN_POINT('Ctrl Pts',(6.46892916984286,-0.687635090018441,5.48549609831644));
#8624=CARTESIAN_POINT('Ctrl Pts',(6.48331906612102,-0.709165727198881,5.08280191239329));
#8625=CARTESIAN_POINT('Ctrl Pts',(6.49774922577713,-0.512546421676701,4.72939501254341));
#8626=CARTESIAN_POINT('Ctrl Pts',(6.50979652059476,-0.216309306596918,4.56725927170696));
#8627=CARTESIAN_POINT('Ctrl Pts',(6.51946444783249,0.0458261865225807,4.54656004710209));
#8628=CARTESIAN_POINT('Ctrl Pts',(6.52670907638838,0.239239492269565,4.58582571736047));
#8629=CARTESIAN_POINT('Ctrl Pts',(6.53399753413874,0.414459889663216,4.67742201785098));
#8630=CARTESIAN_POINT('Ctrl Pts',(6.54121399209174,0.557593347876044,4.81408955941056));
#8631=CARTESIAN_POINT('Ctrl Pts',(6.54677694631745,0.632480164682304,4.94251960028035));
#8632=CARTESIAN_POINT('Ctrl Pts',(6.55027966996043,0.666354521129582,5.03480968054718));
#8633=CARTESIAN_POINT('Ctrl Pts',(6.55215763463341,0.68021361955907,5.08242581586253));
#8634=CARTESIAN_POINT('Ctrl Pts',(6.55432583571746,0.690388365771941,5.13039821778687));
#8635=CARTESIAN_POINT('Ctrl Pts',(6.5558212094319,0.699578648143096,5.19293901702375));
#8636=CARTESIAN_POINT('Ctrl Pts',(6.55961298540583,0.702633425884744,5.28183421164039));
#8637=CARTESIAN_POINT('Ctrl Pts',(6.57151606473466,0.68899661596649,5.41123234210713));
#8638=CARTESIAN_POINT('Ctrl Pts',(6.58803656661797,0.617521153603729,5.63265929180953));
#8639=CARTESIAN_POINT('Ctrl Pts',(6.60958516286006,0.433851269549472,5.83600755874635));
#8640=CARTESIAN_POINT('Ctrl Pts',(6.62973248808607,0.188640588438607,5.94384063293095));
#8641=CARTESIAN_POINT('Ctrl Pts',(6.65043835762877,-0.0772361906896132,
5.98033717006274));
#8642=CARTESIAN_POINT('Ctrl Pts',(6.67615394337537,-0.410324683989954,5.88303784137002));
#8643=CARTESIAN_POINT('Ctrl Pts',(6.70620834369982,-0.677527627921871,5.58106727717635));
#8644=CARTESIAN_POINT('Ctrl Pts',(6.73519774391456,-0.752289167263662,5.20183502623849));
#8645=CARTESIAN_POINT('Ctrl Pts',(6.76319532038265,-0.64086301682906,4.84611638250373));
#8646=CARTESIAN_POINT('Ctrl Pts',(6.79131667826662,-0.371548691224543,4.58557649574375));
#8647=CARTESIAN_POINT('Ctrl Pts',(6.81958651831909,-0.00876747492102148,
4.48516204186951));
#8648=CARTESIAN_POINT('Ctrl Pts',(6.84798778593148,0.359625721045227,4.57071606330109));
#8649=CARTESIAN_POINT('Ctrl Pts',(6.87414419186486,0.619911226291208,4.80259762964785));
#8650=CARTESIAN_POINT('Ctrl Pts',(6.89802078290191,0.743479804719753,5.09040348007126));
#8651=CARTESIAN_POINT('Ctrl Pts',(6.92677090249117,0.75749740723106,5.46842641189442));
#8652=CARTESIAN_POINT('Ctrl Pts',(6.9580730057421,0.540057022180745,5.84196132934458));
#8653=CARTESIAN_POINT('Ctrl Pts',(6.99197236356748,0.126976780802123,6.02565755911728));
#8654=CARTESIAN_POINT('Ctrl Pts',(7.02115368307822,-0.260018076161804,5.99532829292384));
#8655=CARTESIAN_POINT('Ctrl Pts',(7.04435146484917,-0.51904605885336,5.82677537589849));
#8656=CARTESIAN_POINT('Ctrl Pts',(7.06149524329004,-0.653591100025065,5.64982744492753));
#8657=CARTESIAN_POINT('Ctrl Pts',(7.07621223459031,-0.738832249764652,5.47928733188006));
#8658=CARTESIAN_POINT('Ctrl Pts',(7.10202582573893,-0.802074067065736,5.14575072437161));
#8659=CARTESIAN_POINT('Ctrl Pts',(7.1390661714286,-0.614219467641983,4.66923696198742));
#8660=CARTESIAN_POINT('Ctrl Pts',(7.1837708745735,-0.0555595921669689,4.40165548662197));
#8661=CARTESIAN_POINT('Ctrl Pts',(7.22872116331736,0.538653928108292,4.58659194717158));
#8662=CARTESIAN_POINT('Ctrl Pts',(7.27390617378398,0.850481830515366,5.12883749998695));
#8663=CARTESIAN_POINT('Ctrl Pts',(7.31931488180511,0.709264792487632,5.74204700545256));
#8664=CARTESIAN_POINT('Ctrl Pts',(7.35733020712546,0.273950364552491,6.0368560795042));
#8665=CARTESIAN_POINT('Ctrl Pts',(7.38784321768943,-0.127026135903747,6.04956111280713));
#8666=CARTESIAN_POINT('Ctrl Pts',(7.41332435274361,-0.442622948923682,5.93897098677174));
#8667=CARTESIAN_POINT('Ctrl Pts',(7.44141540477827,-0.709991267168369,5.67708175603403));
#8668=CARTESIAN_POINT('Ctrl Pts',(7.47213867876536,-0.829919462138918,5.2858425046348));
#8669=CARTESIAN_POINT('Ctrl Pts',(7.49780365676607,-0.761260797305466,4.9510296020902));
#8670=CARTESIAN_POINT('Ctrl Pts',(7.51837138045615,-0.615435449184283,4.72674446363352));
#8671=CARTESIAN_POINT('Ctrl Pts',(7.53896082495651,-0.41876479320792,4.54455336747707));
#8672=CARTESIAN_POINT('Ctrl Pts',(7.56473451809807,-0.0996332587151797,
4.42005806517321));
#8673=CARTESIAN_POINT('Ctrl Pts',(7.60089474682253,0.379071768057273,4.47943617181632));
#8674=CARTESIAN_POINT('Ctrl Pts',(7.63454183470689,0.719245239568688,4.79620324937939));
#8675=CARTESIAN_POINT('Ctrl Pts',(7.66565790477818,0.822745840976506,5.19215366233993));
#8676=CARTESIAN_POINT('Ctrl Pts',(7.69680539567309,0.778276356479982,5.59852018046501));
#8677=CARTESIAN_POINT('Ctrl Pts',(7.73579429186146,0.441792674687113,6.02084310589315));
#8678=CARTESIAN_POINT('Ctrl Pts',(7.77875200546607,-0.146245218710824,6.10803158972312));
#8679=CARTESIAN_POINT('Ctrl Pts',(7.81784579628705,-0.60534328507275,5.85266747212583));
#8680=CARTESIAN_POINT('Ctrl Pts',(7.85305201517912,-0.833732751184462,5.43911762567102));
#8681=CARTESIAN_POINT('Ctrl Pts',(7.87946834695168,-0.813465377269389,5.08491801220921));
#8682=CARTESIAN_POINT('Ctrl Pts',(7.89708605095421,-0.722929329258105,4.87568490176684));
#8683=CARTESIAN_POINT('Ctrl Pts',(7.90589543440468,-0.663637678579888,4.77837755008365));
#8684=CARTESIAN_POINT('Ctrl Pts',(7.9147052348979,-0.591235696995094,4.69023621557549));
#8685=CARTESIAN_POINT('Ctrl Pts',(7.92840949236335,-0.460683037030015,4.57056164963325));
#8686=CARTESIAN_POINT('Ctrl Pts',(7.95483860408169,-0.15358027728359,4.40642966995394));
#8687=CARTESIAN_POINT('Ctrl Pts',(7.9900782106196,0.331443518324377,4.44333298030211));
#8688=CARTESIAN_POINT('Ctrl Pts',(8.02921328460596,0.723445785656926,4.7953838211401));
#8689=CARTESIAN_POINT('Ctrl Pts',(8.06441280659302,0.854101409558101,5.24877038721031));
#8690=CARTESIAN_POINT('Ctrl Pts',(8.09958701599841,0.723363692643256,5.70295040335949));
#8691=CARTESIAN_POINT('Ctrl Pts',(8.13472653743285,0.371518171835058,6.01720091545639));
#8692=CARTESIAN_POINT('Ctrl Pts',(8.16982494145643,-0.0930948557614484,
6.09627059007613));
#8693=CARTESIAN_POINT('Ctrl Pts',(8.20487462262262,-0.527954026710614,5.91623039165312));
#8694=CARTESIAN_POINT('Ctrl Pts',(8.23986864821332,-0.799991604059477,5.53311237459394));
#8695=CARTESIAN_POINT('Ctrl Pts',(8.27479996206171,-0.826498178537887,5.0648109106924));
#8696=CARTESIAN_POINT('Ctrl Pts',(8.30966173141794,-0.600287084615231,4.65499186138042));
#8697=CARTESIAN_POINT('Ctrl Pts',(8.34444722908088,-0.191633025309102,4.4287921691465));
#8698=CARTESIAN_POINT('Ctrl Pts',(8.37914985495973,0.273621969842747,4.45457183677348));
#8699=CARTESIAN_POINT('Ctrl Pts',(8.41376322201856,0.652891126786519,4.72320094977889));
#8700=CARTESIAN_POINT('Ctrl Pts',(8.44828100386036,0.830672841389853,5.1512269951916));
#8701=CARTESIAN_POINT('Ctrl Pts',(8.48269725010349,0.753725327560749,5.60691060360366));
#8702=CARTESIAN_POINT('Ctrl Pts',(8.51700574767951,0.447197440440791,5.95072247183271));
#8703=CARTESIAN_POINT('Ctrl Pts',(8.55120147675044,0.006056982700166,6.07846248484495));
#8704=CARTESIAN_POINT('Ctrl Pts',(8.5795979930875,-0.360294905244475,5.97323947341581));
#8705=CARTESIAN_POINT('Ctrl Pts',(8.60225515093291,-0.586058809991556,5.78276387703451));
#8706=CARTESIAN_POINT('Ctrl Pts',(8.62361400547052,-0.741423193618978,5.55176886084562));
#8707=CARTESIAN_POINT('Ctrl Pts',(8.6492993869632,-0.80992882190433,5.21659456869169));
#8708=CARTESIAN_POINT('Ctrl Pts',(8.67926816021605,-0.692803381724077,4.83524213198653));
#8709=CARTESIAN_POINT('Ctrl Pts',(8.70663907035742,-0.432425467034378,4.58002223923859));
#8710=CARTESIAN_POINT('Ctrl Pts',(8.73144096068225,-0.125235700856212,4.47256383401499));
#8711=CARTESIAN_POINT('Ctrl Pts',(8.76111878191403,0.264829760437898,4.48474922697656));
#8712=CARTESIAN_POINT('Ctrl Pts',(8.7980518821071,0.687841587709185,4.77102417277571));
#8713=CARTESIAN_POINT('Ctrl Pts',(8.84210282382596,0.824487236093128,5.36617546269049));
#8714=CARTESIAN_POINT('Ctrl Pts',(8.88587709935538,0.522509612312472,5.8912941405695));
#8715=CARTESIAN_POINT('Ctrl Pts',(8.92936793745018,-0.0528251778134879,
6.07023871034585));
#8716=CARTESIAN_POINT('Ctrl Pts',(8.96536876448126,-0.501804297185836,5.85442740754525));
#8717=CARTESIAN_POINT('Ctrl Pts',(8.9940226207963,-0.701513395856217,5.53573257462399));
#8718=CARTESIAN_POINT('Ctrl Pts',(9.02257790961678,-0.774248572961943,5.16726969518564));
#8719=CARTESIAN_POINT('Ctrl Pts',(9.05335063398794,-0.620113902972228,4.77110979993558));
#8720=CARTESIAN_POINT('Ctrl Pts',(9.08629550322002,-0.251166130286266,4.53251972549975));
#8721=CARTESIAN_POINT('Ctrl Pts',(9.11439923362155,0.121398725300332,4.50302942635595));
#8722=CARTESIAN_POINT('Ctrl Pts',(9.14353314968954,0.475903959542619,4.66144572731908));
#8723=CARTESIAN_POINT('Ctrl Pts',(9.17367583697776,0.711198057444889,4.99054851242612));
#8724=CARTESIAN_POINT('Ctrl Pts',(9.20480613272535,0.73620666788718,5.40787508252366));
#8725=CARTESIAN_POINT('Ctrl Pts',(9.23576528071196,0.536473915806161,5.77239779939988));
#8726=CARTESIAN_POINT('Ctrl Pts',(9.2665517671634,0.175449514853214,5.97375916418192));
#8727=CARTESIAN_POINT('Ctrl Pts',(9.29716995899978,-0.235102434914403,5.95230969541478));
#8728=CARTESIAN_POINT('Ctrl Pts',(9.32761122417275,-0.569496724483142,5.71708404420856));
#8729=CARTESIAN_POINT('Ctrl Pts',(9.3578961346874,-0.726661568437755,5.3420504815634));
#8730=CARTESIAN_POINT('Ctrl Pts',(9.3879795972285,-0.660627831242916,4.9431304051231));
#8731=CARTESIAN_POINT('Ctrl Pts',(9.41796225151563,-0.393914336295686,4.64193363228604));
#8732=CARTESIAN_POINT('Ctrl Pts',(9.44267196720143,-0.0739628444132731,
4.5484248269869));
#8733=CARTESIAN_POINT('Ctrl Pts',(9.46256871425264,0.181534913420138,4.58349805707381));
#8734=CARTESIAN_POINT('Ctrl Pts',(9.48193099055251,0.417177415012966,4.68711079083017));
#8735=CARTESIAN_POINT('Ctrl Pts',(9.50264761041058,0.59376362870692,4.8826065496897));
#8736=CARTESIAN_POINT('Ctrl Pts',(9.51853337553614,0.662492027814835,5.09547907660583));
#8737=CARTESIAN_POINT('Ctrl Pts',(9.52998397381837,0.675608484942566,5.22002390776071));
#8738=CARTESIAN_POINT('Ctrl Pts',(9.53360187787314,0.672675837184915,5.30497027631959));
#8739=CARTESIAN_POINT('Ctrl Pts',(9.5350497840785,0.663833420845446,5.3652973078514));
#8740=CARTESIAN_POINT('Ctrl Pts',(9.5371341248435,0.6540363023188,5.41143656975418));
#8741=CARTESIAN_POINT('Ctrl Pts',(9.53893927072564,0.640722782477816,5.45719451112064));
#8742=CARTESIAN_POINT('Ctrl Pts',(9.54230746605352,0.608145268610779,5.54594483650046));
#8743=CARTESIAN_POINT('Ctrl Pts',(9.54765843321268,0.536123532477182,5.66946706886201));
#8744=CARTESIAN_POINT('Ctrl Pts',(9.55460011238389,0.398445319464292,5.8009270775643));
#8745=CARTESIAN_POINT('Ctrl Pts',(9.56161210819828,0.229883573084278,5.88904451423784));
#8746=CARTESIAN_POINT('Ctrl Pts',(9.56858274424492,0.0437972897715726,5.92682689027164));
#8747=CARTESIAN_POINT('Ctrl Pts',(9.57788611107426,-0.208446314292508,5.90690665257042));
#8748=CARTESIAN_POINT('Ctrl Pts',(9.58948273544246,-0.493550672467801,5.75088826678903));
#8749=CARTESIAN_POINT('Ctrl Pts',(9.60337628935687,-0.682895977604234,5.41060732952618));
#8750=CARTESIAN_POINT('Ctrl Pts',(9.61723630723951,-0.662079175861379,5.02289243557709));
#8751=CARTESIAN_POINT('Ctrl Pts',(9.63106693440455,-0.438529006711427,4.70624313314514));
#8752=CARTESIAN_POINT('Ctrl Pts',(9.64486774996197,-0.0814919091113444,
4.55801911650286));
#8753=CARTESIAN_POINT('Ctrl Pts',(9.65863703887208,0.298830266437039,4.62199877125373));
#8754=CARTESIAN_POINT('Ctrl Pts',(9.67238031930236,0.585981516491704,4.87868849034264));
#8755=CARTESIAN_POINT('Ctrl Pts',(9.68151652791651,0.656819784319085,5.12410843764133));
#8756=CARTESIAN_POINT('Ctrl Pts',(9.68608742684445,0.656836403684187,5.24756159158325));
#8757=CARTESIAN_POINT('Ctrl Pts',(6.45926094481572,0.630631645298518,5.25075584038089));
#8758=CARTESIAN_POINT('Ctrl Pts',(6.46365212293046,0.63061567938114,5.36935500462839));
#8759=CARTESIAN_POINT('Ctrl Pts',(6.47241635726032,0.562620260489693,5.60485419658667));
#8760=CARTESIAN_POINT('Ctrl Pts',(6.48558625248065,0.287416865857649,5.85077154136491));
#8761=CARTESIAN_POINT('Ctrl Pts',(6.49876139799279,-0.0766327666807152,
5.91202548479231));
#8762=CARTESIAN_POINT('Ctrl Pts',(6.51195067642553,-0.417708947598931,5.77004045811818));
#8763=CARTESIAN_POINT('Ctrl Pts',(6.52514978293253,-0.631222811810323,5.46797327754339));
#8764=CARTESIAN_POINT('Ctrl Pts',(6.53835654602454,-0.650891881237755,5.09827400825114));
#8765=CARTESIAN_POINT('Ctrl Pts',(6.55158109914582,-0.470586715770342,4.77436995516259));
#8766=CARTESIAN_POINT('Ctrl Pts',(6.56260333534973,-0.199433661178286,4.62604524416983));
#8767=CARTESIAN_POINT('Ctrl Pts',(6.571441254142,0.0402205362572792,4.60713511034868));
#8768=CARTESIAN_POINT('Ctrl Pts',(6.57805870994194,0.216917555899971,4.64301726701627));
#8769=CARTESIAN_POINT('Ctrl Pts',(6.58471156897691,0.376868484589112,4.7266438859889));
#8770=CARTESIAN_POINT('Ctrl Pts',(6.59129368162691,0.507448482818788,4.8513301406675));
#8771=CARTESIAN_POINT('Ctrl Pts',(6.59636476168569,0.575693818909383,4.96841258612528));
#8772=CARTESIAN_POINT('Ctrl Pts',(6.59955449451534,0.606568241636653,5.05249416408791));
#8773=CARTESIAN_POINT('Ctrl Pts',(6.60126044558016,0.619113836374534,5.09569120029176));
#8774=CARTESIAN_POINT('Ctrl Pts',(6.60323132681257,0.628456403477267,5.13943435527507));
#8775=CARTESIAN_POINT('Ctrl Pts',(6.6046510101575,0.636856623460891,5.19748854771694));
#8776=CARTESIAN_POINT('Ctrl Pts',(6.6079401285395,0.639609543705504,5.27534803811019));
#8777=CARTESIAN_POINT('Ctrl Pts',(6.61879883010074,0.627183581911554,5.39376860016358));
#8778=CARTESIAN_POINT('Ctrl Pts',(6.63383329382943,0.562134630004875,5.59501981359328));
#8779=CARTESIAN_POINT('Ctrl Pts',(6.65338763271038,0.395327976071264,5.77969125230577));
#8780=CARTESIAN_POINT('Ctrl Pts',(6.67164286743441,0.173140595239862,5.87732250405325));
#8781=CARTESIAN_POINT('Ctrl Pts',(6.69038342521688,-0.0675226512948717,
5.91034880637455));
#8782=CARTESIAN_POINT('Ctrl Pts',(6.71361724126403,-0.368479602326163,5.82230340539203));
#8783=CARTESIAN_POINT('Ctrl Pts',(6.74072150009791,-0.60939880453155,5.54988058932266));
#8784=CARTESIAN_POINT('Ctrl Pts',(6.76682335000588,-0.676647905208886,5.2083655360096));
#8785=CARTESIAN_POINT('Ctrl Pts',(6.79199917821714,-0.576386826274553,4.88848696990566));
#8786=CARTESIAN_POINT('Ctrl Pts',(6.81725659668747,-0.334439787297777,4.65449398609593));
#8787=CARTESIAN_POINT('Ctrl Pts',(6.84262441363562,-0.00888238488552531,
4.56442303985172));
#8788=CARTESIAN_POINT('Ctrl Pts',(6.86808919715576,0.321423032235318,4.64116571674426));
#8789=CARTESIAN_POINT('Ctrl Pts',(6.89152618201979,0.554634130589795,4.84896006600901));
#8790=CARTESIAN_POINT('Ctrl Pts',(6.91291206541523,0.665305615860708,5.10674832578124));
#8791=CARTESIAN_POINT('Ctrl Pts',(6.93865672617456,0.677845262595485,5.44525276052196));
#8792=CARTESIAN_POINT('Ctrl Pts',(6.9666802969137,0.483167022914325,5.77965370335718));
#8793=CARTESIAN_POINT('Ctrl Pts',(6.99703059331053,0.113343713819975,5.94411784378224));
#8794=CARTESIAN_POINT('Ctrl Pts',(7.0231623426855,-0.23320446349144,5.91696869874648));
#8795=CARTESIAN_POINT('Ctrl Pts',(7.04394514044647,-0.465252901929868,5.76598107103288));
#8796=CARTESIAN_POINT('Ctrl Pts',(7.05930843146434,-0.585824133571807,5.60741425568615));
#8797=CARTESIAN_POINT('Ctrl Pts',(7.07250016431883,-0.66222795488503,5.45455360274052));
#8798=CARTESIAN_POINT('Ctrl Pts',(7.09564685442722,-0.718945508527952,5.15549592008938));
#8799=CARTESIAN_POINT('Ctrl Pts',(7.12889075561355,-0.550454960488801,4.72782148892568));
#8800=CARTESIAN_POINT('Ctrl Pts',(7.16907295422903,-0.0484319759876638,
4.48718062663814));
#8801=CARTESIAN_POINT('Ctrl Pts',(7.20954974681085,0.486652722950244,4.65350202049014));
#8802=CARTESIAN_POINT('Ctrl Pts',(7.25032543086917,0.768219032236227,5.14265428374656));
#8803=CARTESIAN_POINT('Ctrl Pts',(7.29140272492947,0.640759617553892,5.69737175715812));
#8804=CARTESIAN_POINT('Ctrl Pts',(7.32588776974505,0.246065794644022,5.96496491665055));
#8805=CARTESIAN_POINT('Ctrl Pts',(7.35362729609519,-0.118440598074296,5.97657459585275));
#8806=CARTESIAN_POINT('Ctrl Pts',(7.37682808694136,-0.405776263850554,5.87592416000432));
#8807=CARTESIAN_POINT('Ctrl Pts',(7.40246011243668,-0.649742181768781,5.63708400277588));
#8808=CARTESIAN_POINT('Ctrl Pts',(7.43055732482948,-0.759491260397883,5.27939247550575));
#8809=CARTESIAN_POINT('Ctrl Pts',(7.45408328696561,-0.696658442318083,4.97251220294606));
#8810=CARTESIAN_POINT('Ctrl Pts',(7.47297033777351,-0.562772704954616,4.76656163926831));
#8811=CARTESIAN_POINT('Ctrl Pts',(7.49190239095096,-0.381972617311867,4.59904546261976));
#8812=CARTESIAN_POINT('Ctrl Pts',(7.51565348005123,-0.0879986165622313,
4.48426496479248));
#8813=CARTESIAN_POINT('Ctrl Pts',(7.54905384695099,0.354151719711531,4.53895015859063));
#8814=CARTESIAN_POINT('Ctrl Pts',(7.58025012786886,0.669708281866875,4.83233675359967));
#8815=CARTESIAN_POINT('Ctrl Pts',(7.60918908886255,0.766049363842592,5.20056109169432));
#8816=CARTESIAN_POINT('Ctrl Pts',(7.63822532543653,0.724677250086816,5.57929734522926));
#8817=CARTESIAN_POINT('Ctrl Pts',(7.67470077570181,0.410318385521739,5.97456130664251));
#8818=CARTESIAN_POINT('Ctrl Pts',(7.71507638215079,-0.142205641163269,6.05698865126465));
#8819=CARTESIAN_POINT('Ctrl Pts',(7.75197857351751,-0.575616781704155,5.81621148710719));
#8820=CARTESIAN_POINT('Ctrl Pts',(7.7853417233448,-0.792188660547873,5.42454893449295));
#8821=CARTESIAN_POINT('Ctrl Pts',(7.81047387915203,-0.773098565169157,5.08768447811596));
#8822=CARTESIAN_POINT('Ctrl Pts',(7.82726838473859,-0.686808914769296,4.88823688066732));
#8823=CARTESIAN_POINT('Ctrl Pts',(7.835674306709,-0.630239891545833,4.7953931849875));
#8824=CARTESIAN_POINT('Ctrl Pts',(7.84408881413366,-0.561096499472987,4.71120959694044));
#8825=CARTESIAN_POINT('Ctrl Pts',(7.85719169921437,-0.436283161532637,4.59679757004653));
#8826=CARTESIAN_POINT('Ctrl Pts',(7.88250981486252,-0.142222857964216,4.43951581665192));
#8827=CARTESIAN_POINT('Ctrl Pts',(7.91639613701036,0.324197674501624,4.47456645604085));
#8828=CARTESIAN_POINT('Ctrl Pts',(7.95421610770856,0.703178520684008,4.8144802854019));
#8829=CARTESIAN_POINT('Ctrl Pts',(7.98837804458697,0.83019336282416,5.25430147573914));
#8830=CARTESIAN_POINT('Ctrl Pts',(8.02265345717082,0.703100029192506,5.69683666807885));
#8831=CARTESIAN_POINT('Ctrl Pts',(8.05703932219342,0.359082622660234,6.00447747470694));
#8832=CARTESIAN_POINT('Ctrl Pts',(8.09152885121967,-0.0973054214259819,
6.08243030040749));
#8833=CARTESIAN_POINT('Ctrl Pts',(8.12611659734114,-0.526430256741482,5.90506932981871));
#8834=CARTESIAN_POINT('Ctrl Pts',(8.16079619608074,-0.796185325416799,5.5256490871169));
#8835=CARTESIAN_POINT('Ctrl Pts',(8.19556142276615,-0.822839939891373,5.05970301502219));
#8836=CARTESIAN_POINT('Ctrl Pts',(8.2304057358346,-0.597042136063547,4.65004920673372));
#8837=CARTESIAN_POINT('Ctrl Pts',(8.26532250261526,-0.187078096730767,4.42280111950569));
#8838=CARTESIAN_POINT('Ctrl Pts',(8.30030493712832,0.281835625706235,4.44849940120078));
#8839=CARTESIAN_POINT('Ctrl Pts',(8.335346094925,0.665868121349874,4.72015532769358));
#8840=CARTESIAN_POINT('Ctrl Pts',(8.37043908067028,0.846830207518658,5.15510382746606));
#8841=CARTESIAN_POINT('Ctrl Pts',(8.40557652216204,0.76856474297763,5.62027880248826));
#8842=CARTESIAN_POINT('Ctrl Pts',(8.44075186874733,0.454573489708275,5.9728735479694));
#8843=CARTESIAN_POINT('Ctrl Pts',(8.47595655163873,0.000592216545345121,
6.10462424972125));
#8844=CARTESIAN_POINT('Ctrl Pts',(8.50531485448479,-0.378126834876055,5.99608292083659));
#8845=CARTESIAN_POINT('Ctrl Pts',(8.52880549491824,-0.61220217773172,5.79865133938525));
#8846=CARTESIAN_POINT('Ctrl Pts',(8.55099425377555,-0.773619699372566,5.55873173979293));
#8847=CARTESIAN_POINT('Ctrl Pts',(8.57776180819305,-0.845133662349741,5.20958202612232));
#8848=CARTESIAN_POINT('Ctrl Pts',(8.60909324987135,-0.722872864715742,4.81086604976394));
#8849=CARTESIAN_POINT('Ctrl Pts',(8.63781260447889,-0.449832178475452,4.54300286426828));
#8850=CARTESIAN_POINT('Ctrl Pts',(8.66391301341504,-0.126615872418881,4.42985501290241));
#8851=CARTESIAN_POINT('Ctrl Pts',(8.69522182105708,0.284827089964824,4.44259765149754));
#8852=CARTESIAN_POINT('Ctrl Pts',(8.73433751096835,0.733021979172566,4.74531837229694));
#8853=CARTESIAN_POINT('Ctrl Pts',(8.78121985601859,0.879026849711619,5.37848771966574));
#8854=CARTESIAN_POINT('Ctrl Pts',(8.82802879092876,0.556658256670406,5.94020744536304));
#8855=CARTESIAN_POINT('Ctrl Pts',(8.87474682574646,-0.0611139932480479,
6.13293868276154));
#8856=CARTESIAN_POINT('Ctrl Pts',(8.913590527633,-0.545669664063004,5.90050291517835));
#8857=CARTESIAN_POINT('Ctrl Pts',(8.94460190831635,-0.761866942586277,5.55563994385839));
#8858=CARTESIAN_POINT('Ctrl Pts',(8.97556820450398,-0.840825162899319,5.15613185120987));
#8859=CARTESIAN_POINT('Ctrl Pts',(9.00904197636457,-0.673477940739932,4.72513624475881));
#8860=CARTESIAN_POINT('Ctrl Pts',(9.04498768824832,-0.271018916657287,4.46467281490372));
#8861=CARTESIAN_POINT('Ctrl Pts',(9.07572502891324,0.136431921301358,4.4323095041422));
#8862=CARTESIAN_POINT('Ctrl Pts',(9.1076623520104,0.525083004968427,4.60584001971559));
#8863=CARTESIAN_POINT('Ctrl Pts',(9.14078441660845,0.783740757738325,4.96735319118576));
#8864=CARTESIAN_POINT('Ctrl Pts',(9.17506955917779,0.811435257145466,5.42693255065578));
#8865=CARTESIAN_POINT('Ctrl Pts',(9.20923929276318,0.591126060121817,5.82930504824957));
#8866=CARTESIAN_POINT('Ctrl Pts',(9.2432856375487,0.191952178313332,6.05209191391443));
#8867=CARTESIAN_POINT('Ctrl Pts',(9.27720741279787,-0.262891492169015,6.02844633536177));
#8868=CARTESIAN_POINT('Ctrl Pts',(9.31098858952086,-0.63403272803984,5.76750123179495));
#8869=CARTESIAN_POINT('Ctrl Pts',(9.34464578869081,-0.808786198417316,5.35074288886772));
#8870=CARTESIAN_POINT('Ctrl Pts',(9.37812199499848,-0.735387937206534,4.90681109950957));
#8871=CARTESIAN_POINT('Ctrl Pts',(9.41152322842209,-0.438313831815708,4.5712184418284));
#8872=CARTESIAN_POINT('Ctrl Pts',(9.43907484027071,-0.0815663109302454,
4.4669012937477));
#8873=CARTESIAN_POINT('Ctrl Pts',(9.4612729336839,0.203489644522288,4.50602296930772));
#8874=CARTESIAN_POINT('Ctrl Pts',(9.48288145933666,0.466474214399761,4.62164830317789));
#8875=CARTESIAN_POINT('Ctrl Pts',(9.50600861598851,0.663637471981693,4.83989009112341));
#8876=CARTESIAN_POINT('Ctrl Pts',(9.5237504983284,0.740394735416907,5.07762350734759));
#8877=CARTESIAN_POINT('Ctrl Pts',(9.53653973758647,0.755044636738244,5.21674586453469));
#8878=CARTESIAN_POINT('Ctrl Pts',(9.54057094671748,0.75177110427318,5.31144642435382));
#8879=CARTESIAN_POINT('Ctrl Pts',(9.54219323251979,0.741887195738976,5.37894319660566));
#8880=CARTESIAN_POINT('Ctrl Pts',(9.5445220671336,0.730934116011717,5.43050504199544));
#8881=CARTESIAN_POINT('Ctrl Pts',(9.54653892088636,0.71606192719596,5.48162749166749));
#8882=CARTESIAN_POINT('Ctrl Pts',(9.55030275855579,0.679655812307881,5.58080645949484));
#8883=CARTESIAN_POINT('Ctrl Pts',(9.55628190241597,0.599176010120261,5.71884228830231));
#8884=CARTESIAN_POINT('Ctrl Pts',(9.56403888456,0.445318424533598,5.86575289756921));
#8885=CARTESIAN_POINT('Ctrl Pts',(9.57187432376913,0.256949209836898,5.96422582543611));
#8886=CARTESIAN_POINT('Ctrl Pts',(9.57966347320304,0.0489975353055775,6.00644848836681));
#8887=CARTESIAN_POINT('Ctrl Pts',(9.59005920748721,-0.232880677765524,5.98418877373988));
#8888=CARTESIAN_POINT('Ctrl Pts',(9.60301490728257,-0.551448605271625,5.809856277591));
#8889=CARTESIAN_POINT('Ctrl Pts',(9.6185356227464,-0.762994742028112,5.42967706691061));
#8890=CARTESIAN_POINT('Ctrl Pts',(9.63401589798779,-0.739733408664225,4.99657949737655));
#8891=CARTESIAN_POINT('Ctrl Pts',(9.64945947119682,-0.490079410801249,4.64296802543169));
#8892=CARTESIAN_POINT('Ctrl Pts',(9.66486611496518,-0.0914480651653445,
4.47748174052505));
#8893=CARTESIAN_POINT('Ctrl Pts',(9.68023447346001,0.333029170036261,4.5489404444483));
#8894=CARTESIAN_POINT('Ctrl Pts',(9.69556462598151,0.653376293098328,4.83529182895193));
#8895=CARTESIAN_POINT('Ctrl Pts',(9.70575657704672,0.732335431233298,5.10911134118588));
#8896=CARTESIAN_POINT('Ctrl Pts',(9.71084842832256,0.732353944732881,5.24663464006324));
#8897=CARTESIAN_POINT('Ctrl Pts',(6.53677890889994,0.648308344097312,5.24788808861526));
#8898=CARTESIAN_POINT('Ctrl Pts',(6.54128841999409,0.648291947932169,5.36968324994926));
#8899=CARTESIAN_POINT('Ctrl Pts',(6.55029072386857,0.578366883190402,5.61148400116062));
#8900=CARTESIAN_POINT('Ctrl Pts',(6.56377552959342,0.296488302798292,5.86313472695387));
#8901=CARTESIAN_POINT('Ctrl Pts',(6.57723486151276,-0.0753487981176404,
5.92558903258212));
#8902=CARTESIAN_POINT('Ctrl Pts',(6.59067201260385,-0.422743869195993,5.78083317969924));
#8903=CARTESIAN_POINT('Ctrl Pts',(6.60408642445702,-0.639583194854741,5.47384153684459));
#8904=CARTESIAN_POINT('Ctrl Pts',(6.61747718701865,-0.659388633790789,5.09914333460697));
#8905=CARTESIAN_POINT('Ctrl Pts',(6.63084921534714,-0.477002675415156,4.77178831487133));
#8906=CARTESIAN_POINT('Ctrl Pts',(6.64196797156513,-0.203535776818503,4.62233154714453));
#8907=CARTESIAN_POINT('Ctrl Pts',(6.65086270156841,0.0376212461558179,4.60332808393359));
#8908=CARTESIAN_POINT('Ctrl Pts',(6.65751436882366,0.215206656454501,4.63940682661395));
#8909=CARTESIAN_POINT('Ctrl Pts',(6.66419350349961,0.375739235616664,4.72336011101286));
#8910=CARTESIAN_POINT('Ctrl Pts',(6.67079173242759,0.506648525281715,4.84836014585996));
#8911=CARTESIAN_POINT('Ctrl Pts',(6.67587168733797,0.574942135378562,4.96558591415989));
#8912=CARTESIAN_POINT('Ctrl Pts',(6.67905830408769,0.605836587356559,5.0496479041938));
#8913=CARTESIAN_POINT('Ctrl Pts',(6.68075445132886,0.61822311366418,5.09247873674454));
#8914=CARTESIAN_POINT('Ctrl Pts',(6.68271633522742,0.627705254751127,5.13628244164802));
#8915=CARTESIAN_POINT('Ctrl Pts',(6.68424751516306,0.636157930364232,5.19641973994768));
#8916=CARTESIAN_POINT('Ctrl Pts',(6.68721504263871,0.638850758901545,5.26817630302783));
#8917=CARTESIAN_POINT('Ctrl Pts',(6.6980886411611,0.626432492962911,5.38747198490893));
#8918=CARTESIAN_POINT('Ctrl Pts',(6.7130742817883,0.561598102708803,5.58757297033252));
#8919=CARTESIAN_POINT('Ctrl Pts',(6.73247121050942,0.395939555636536,5.77092466279022));
#8920=CARTESIAN_POINT('Ctrl Pts',(6.75050076668837,0.176511931668019,5.86718938307879));
#8921=CARTESIAN_POINT('Ctrl Pts',(6.76896343885092,-0.0605850594853099,
5.89971030240676));
#8922=CARTESIAN_POINT('Ctrl Pts',(6.79176314959733,-0.35582242285045,5.81305067264655));
#8923=CARTESIAN_POINT('Ctrl Pts',(6.81822260673932,-0.590783555636119,5.54697381679167));
#8924=CARTESIAN_POINT('Ctrl Pts',(6.84357792410812,-0.655910626230322,5.21520740643816));
#8925=CARTESIAN_POINT('Ctrl Pts',(6.86792311414774,-0.558797745057059,4.90596294050986));
#8926=CARTESIAN_POINT('Ctrl Pts',(6.89223845562662,-0.325774686137532,4.68084210219441));
#8927=CARTESIAN_POINT('Ctrl Pts',(6.91655009079728,-0.0137382982285809,
4.59469205345031));
#8928=CARTESIAN_POINT('Ctrl Pts',(6.94085000037151,0.301406716506307,4.66808590961898));
#8929=CARTESIAN_POINT('Ctrl Pts',(6.96312145304551,0.522894871174355,4.86564283981171));
#8930=CARTESIAN_POINT('Ctrl Pts',(6.98336932148207,0.627613721193077,5.10972341863593));
#8931=CARTESIAN_POINT('Ctrl Pts',(7.00767034974037,0.639345410745925,5.42926415376025));
#8932=CARTESIAN_POINT('Ctrl Pts',(7.0340061377139,0.456096194913984,5.74332463138044));
#8933=CARTESIAN_POINT('Ctrl Pts',(7.06239212271459,0.110146516358368,5.89696458325904));
#8934=CARTESIAN_POINT('Ctrl Pts',(7.08674403780546,-0.212777772472184,5.87153444736802));
#8935=CARTESIAN_POINT('Ctrl Pts',(7.10604298073846,-0.428203986860686,5.73123639550283));
#8936=CARTESIAN_POINT('Ctrl Pts',(7.1202763794347,-0.539896968044911,5.58432836902718));
#8937=CARTESIAN_POINT('Ctrl Pts',(7.13248259304633,-0.610589669953036,5.44288429135274));
#8938=CARTESIAN_POINT('Ctrl Pts',(7.15386080729459,-0.662907145870833,5.16664121175135));
#8939=CARTESIAN_POINT('Ctrl Pts',(7.18445524346917,-0.507518708932404,4.77315870520267));
#8940=CARTESIAN_POINT('Ctrl Pts',(7.2212730060695,-0.0473329540045874,4.55302086919988));
#8941=CARTESIAN_POINT('Ctrl Pts',(7.25821128490183,0.440889209665914,4.70515440715441));
#8942=CARTESIAN_POINT('Ctrl Pts',(7.29528590651588,0.696637153045051,5.15010859139779));
#8943=CARTESIAN_POINT('Ctrl Pts',(7.332512739643,0.58082551013422,5.65279628754744));
#8944=CARTESIAN_POINT('Ctrl Pts',(7.3636735148449,0.224022453087409,5.89445423698418));
#8945=CARTESIAN_POINT('Ctrl Pts',(7.38869394277869,-0.104770142311705,5.9048883954555));
#8946=CARTESIAN_POINT('Ctrl Pts',(7.4095969054791,-0.363665133915886,5.81417857686521));
#8947=CARTESIAN_POINT('Ctrl Pts',(7.43265719036872,-0.583169551820776,5.59922290709689));
#8948=CARTESIAN_POINT('Ctrl Pts',(7.45790499477554,-0.681772872980722,5.27773207396749));
#8949=CARTESIAN_POINT('Ctrl Pts',(7.47902438387107,-0.625327749884945,5.00220880580607));
#8950=CARTESIAN_POINT('Ctrl Pts',(7.49596985369807,-0.505194085748851,4.81741578549234));
#8951=CARTESIAN_POINT('Ctrl Pts',(7.51294825933135,-0.343029342279038,4.66716861489283));
#8952=CARTESIAN_POINT('Ctrl Pts',(7.53423229204698,-0.0795149396536471,
4.56430162846121));
#8953=CARTESIAN_POINT('Ctrl Pts',(7.56415795707461,0.316651231938915,4.61331432755186));
#8954=CARTESIAN_POINT('Ctrl Pts',(7.59208894080855,0.599222510850577,4.8760718061598));
#8955=CARTESIAN_POINT('Ctrl Pts',(7.61800089328846,0.685499071631382,5.20580221532286));
#8956=CARTESIAN_POINT('Ctrl Pts',(7.64399762025679,0.648452480668231,5.5449492628021));
#8957=CARTESIAN_POINT('Ctrl Pts',(7.6766558308975,0.366948218153944,5.89895940428666));
#8958=CARTESIAN_POINT('Ctrl Pts',(7.71283041368628,-0.128170599844781,5.97289577401557));
#8959=CARTESIAN_POINT('Ctrl Pts',(7.74591955350209,-0.516915920064396,5.75700818829182));
#8960=CARTESIAN_POINT('Ctrl Pts',(7.77585687382348,-0.711357071237054,5.4054746092851));
#8961=CARTESIAN_POINT('Ctrl Pts',(7.79843023324687,-0.694254716447698,5.10278765610887));
#8962=CARTESIAN_POINT('Ctrl Pts',(7.81353402254503,-0.616644573867706,4.92340025453556));
#8963=CARTESIAN_POINT('Ctrl Pts',(7.82109624603377,-0.565750095788821,4.83986786624699));
#8964=CARTESIAN_POINT('Ctrl Pts',(7.82866883860509,-0.503521173252006,4.76409997528913));
#8965=CARTESIAN_POINT('Ctrl Pts',(7.84046426369671,-0.391150332502584,4.66109170486198));
#8966=CARTESIAN_POINT('Ctrl Pts',(7.86326838969153,-0.126269457842156,4.51937164453054));
#8967=CARTESIAN_POINT('Ctrl Pts',(7.89384459534472,0.294624621968566,4.55083813829548));
#8968=CARTESIAN_POINT('Ctrl Pts',(7.92803343879433,0.637390764050739,4.85808320500068));
#8969=CARTESIAN_POINT('Ctrl Pts',(7.95897115106736,0.752557991506694,5.25650008748354));
#8970=CARTESIAN_POINT('Ctrl Pts',(7.99008150777189,0.637292674479974,5.6583098830911));
#8971=CARTESIAN_POINT('Ctrl Pts',(8.02136268813123,0.324328340887489,5.93835687143453));
#8972=CARTESIAN_POINT('Ctrl Pts',(8.05281552085117,-0.0919668369256177,
6.0096089960033));
#8973=CARTESIAN_POINT('Ctrl Pts',(8.08443922850855,-0.484488081008684,5.84754699761468));
#8974=CARTESIAN_POINT('Ctrl Pts',(8.11623331579657,-0.732001743146474,5.49969950716172));
#8975=CARTESIAN_POINT('Ctrl Pts',(8.14819672239933,-0.756691626879712,5.07120150721029));
#8976=CARTESIAN_POINT('Ctrl Pts',(8.18032818682298,-0.548581427785167,4.69325383595664));
#8977=CARTESIAN_POINT('Ctrl Pts',(8.21262609933926,-0.169361160919892,4.48282710725417));
#8978=CARTESIAN_POINT('Ctrl Pts',(8.24508852965908,0.265897639458044,4.50648066670812));
#8979=CARTESIAN_POINT('Ctrl Pts',(8.27771329285446,0.623659903118161,4.7592998152198));
#8980=CARTESIAN_POINT('Ctrl Pts',(8.31049776406179,0.792961734420276,5.16566132423459));
#8981=CARTESIAN_POINT('Ctrl Pts',(8.34343929891669,0.719787629314293,5.60191531751229));
#8982=CARTESIAN_POINT('Ctrl Pts',(8.3765342962972,0.424457038652123,5.9339034705343));
#8983=CARTESIAN_POINT('Ctrl Pts',(8.40978030794087,-0.00430578935872142,
6.05858175740242));
#8984=CARTESIAN_POINT('Ctrl Pts',(8.43760606022993,-0.363432150149208,5.9558615895779));
#8985=CARTESIAN_POINT('Ctrl Pts',(8.45994080550056,-0.58605591073669,5.76814595608163));
#8986=CARTESIAN_POINT('Ctrl Pts',(8.48107939877234,-0.73987545479849,5.53958299989996));
#8987=CARTESIAN_POINT('Ctrl Pts',(8.5066384857038,-0.808346850487237,5.20610228318772));
#8988=CARTESIAN_POINT('Ctrl Pts',(8.53667295472767,-0.691293438814756,4.82379987835255));
#8989=CARTESIAN_POINT('Ctrl Pts',(8.56429709374726,-0.42873318070134,4.56597536887464));
#8990=CARTESIAN_POINT('Ctrl Pts',(8.58948347459684,-0.116793468377635,4.45670239484369));
#8991=CARTESIAN_POINT('Ctrl Pts',(8.61978105797819,0.281366713802581,4.46891907801678));
#8992=CARTESIAN_POINT('Ctrl Pts',(8.65778272897614,0.717169109368427,4.76263678021251));
#8993=CARTESIAN_POINT('Ctrl Pts',(8.70358396899606,0.86049511964979,5.38117382901366));
#8994=CARTESIAN_POINT('Ctrl Pts',(8.74957058756189,0.544301662499638,5.93347229333488));
#8995=CARTESIAN_POINT('Ctrl Pts',(8.79572865872733,-0.0659692059206899,
6.12458004624303));
#8996=CARTESIAN_POINT('Ctrl Pts',(8.83432310014984,-0.547772509862173,5.89408580556368));
#8997=CARTESIAN_POINT('Ctrl Pts',(8.86527036286416,-0.763656389723532,5.54991022181832));
#8998=CARTESIAN_POINT('Ctrl Pts',(8.89626292036845,-0.842796411694417,5.15009597609929));
#8999=CARTESIAN_POINT('Ctrl Pts',(8.92990401221682,-0.675022169192827,4.71671716418602));
#9000=CARTESIAN_POINT('Ctrl Pts',(8.9662054975265,-0.26866399657737,4.4534420925465));
#9001=CARTESIAN_POINT('Ctrl Pts',(8.99736409597451,0.144379983188026,4.4204521703534));
#9002=CARTESIAN_POINT('Ctrl Pts',(9.02986103725035,0.539947482583334,4.59684672007972));
#9003=CARTESIAN_POINT('Ctrl Pts',(9.06369328425281,0.804398444941881,4.96601673371496));
#9004=CARTESIAN_POINT('Ctrl Pts',(9.09886203052067,0.833075652533933,5.43747935159163));
#9005=CARTESIAN_POINT('Ctrl Pts',(9.13405836073647,0.606349827859166,5.8521164848996));
#9006=CARTESIAN_POINT('Ctrl Pts',(9.16927256307506,0.193565787562334,6.08279802034468));
#9007=CARTESIAN_POINT('Ctrl Pts',(9.20450120399963,-0.278862713204365,6.05849885410467));
#9008=CARTESIAN_POINT('Ctrl Pts',(9.23972501673659,-0.666042337314815,5.78659268801242));
#9009=CARTESIAN_POINT('Ctrl Pts',(9.27495928577355,-0.849238451522511,5.35036898675046));
#9010=CARTESIAN_POINT('Ctrl Pts',(9.3101402023598,-0.77235128088339,4.88373310289506));
#9011=CARTESIAN_POINT('Ctrl Pts',(9.34537826519511,-0.459114700993423,4.52949905625442));
#9012=CARTESIAN_POINT('Ctrl Pts',(9.37455217501767,-0.0813826670684427,
4.41879392741861));
#9013=CARTESIAN_POINT('Ctrl Pts',(9.39812483474283,0.221347040696434,4.46032370541366));
#9014=CARTESIAN_POINT('Ctrl Pts',(9.42111143712525,0.501106191970378,4.58320002284348));
#9015=CARTESIAN_POINT('Ctrl Pts',(9.44577928522819,0.711600998294542,4.81615110634447));
#9016=CARTESIAN_POINT('Ctrl Pts',(9.46476901472948,0.793754078120072,5.07020874147712));
#9017=CARTESIAN_POINT('Ctrl Pts',(9.4784973521178,0.809459762090862,5.22012003835188));
#9018=CARTESIAN_POINT('Ctrl Pts',(9.48256220237874,0.80599714391194,5.31678427772113));
#9019=CARTESIAN_POINT('Ctrl Pts',(9.48439284136576,0.79535027000064,5.39088618359879));
#9020=CARTESIAN_POINT('Ctrl Pts',(9.4868839869042,0.783486446136706,5.44625321444756));
#9021=CARTESIAN_POINT('Ctrl Pts',(9.48903979693529,0.76765908397162,5.50080528896331));
#9022=CARTESIAN_POINT('Ctrl Pts',(9.49307526895426,0.728584239469491,5.60719555343428));
#9023=CARTESIAN_POINT('Ctrl Pts',(9.49949589017351,0.642208233985685,5.75539627308332));
#9024=CARTESIAN_POINT('Ctrl Pts',(9.50782995020485,0.476882658707867,5.91325735933798));
#9025=CARTESIAN_POINT('Ctrl Pts',(9.51625602332589,0.274333603849002,6.0191596722041));
#9026=CARTESIAN_POINT('Ctrl Pts',(9.52463871614711,0.0505347313054355,6.06461215503176));
#9027=CARTESIAN_POINT('Ctrl Pts',(9.53583562734331,-0.253057457619835,6.04065652197636));
#9028=CARTESIAN_POINT('Ctrl Pts',(9.5498071049154,-0.596622179197612,5.85274547177686));
#9029=CARTESIAN_POINT('Ctrl Pts',(9.56657059349091,-0.825178633194954,5.44220828219499));
#9030=CARTESIAN_POINT('Ctrl Pts',(9.58331580941746,-0.800115741031158,4.97374519727449));
#9031=CARTESIAN_POINT('Ctrl Pts',(9.60004749969833,-0.529743331948014,4.59064885817877));
#9032=CARTESIAN_POINT('Ctrl Pts',(9.61676192682012,-0.0973151100553377,
4.41101912125671));
#9033=CARTESIAN_POINT('Ctrl Pts',(9.63346072597428,0.363869421061874,4.48860536541958));
#9034=CARTESIAN_POINT('Ctrl Pts',(9.65013784702028,0.712465653120617,4.80001782474214));
#9035=CARTESIAN_POINT('Ctrl Pts',(9.66124801098291,0.79856285759502,5.09847089746305));
#9036=CARTESIAN_POINT('Ctrl Pts',(9.66679389193444,0.798583021904447,5.24825685984085));
#9037=CARTESIAN_POINT('Ctrl Pts',(6.55985766373767,0.695773542681336,5.24703997894806));
#9038=CARTESIAN_POINT('Ctrl Pts',(6.56469408527635,0.695755957900061,5.37766450326637));
#9039=CARTESIAN_POINT('Ctrl Pts',(6.57435500114752,0.620735066792372,5.6371846277021));
#9040=CARTESIAN_POINT('Ctrl Pts',(6.58881199472521,0.318467016967517,5.90695568638057));
#9041=CARTESIAN_POINT('Ctrl Pts',(6.60323442988062,-0.0799854836502877,
5.97386387712081));
#9042=CARTESIAN_POINT('Ctrl Pts',(6.61762277610453,-0.451981525128358,5.81879973852038));
#9043=CARTESIAN_POINT('Ctrl Pts',(6.63197659243013,-0.68398248083499,5.49026587240634));
#9044=CARTESIAN_POINT('Ctrl Pts',(6.64629279495561,-0.705102229235322,5.08960601326795));
#9045=CARTESIAN_POINT('Ctrl Pts',(6.66057898517367,-0.510181991891156,4.73986607438693));
#9046=CARTESIAN_POINT('Ctrl Pts',(6.6724472572393,-0.218209859199235,4.58035203049584));
#9047=CARTESIAN_POINT('Ctrl Pts',(6.68193687531017,0.039087393851036,4.56008746412766));
#9048=CARTESIAN_POINT('Ctrl Pts',(6.68903012532506,0.228476658021195,4.59857220869176));
#9049=CARTESIAN_POINT('Ctrl Pts',(6.6961496976064,0.399596133977577,4.68807212672819));
#9050=CARTESIAN_POINT('Ctrl Pts',(6.7031795050705,0.539084893132951,4.8212679598734));
#9051=CARTESIAN_POINT('Ctrl Pts',(6.70858995882373,0.611801754599193,4.94611855978549));
#9052=CARTESIAN_POINT('Ctrl Pts',(6.71198117635767,0.644700212006901,5.03560603181988));
#9053=CARTESIAN_POINT('Ctrl Pts',(6.71378304218766,0.657824365352093,5.08106104415238));
#9054=CARTESIAN_POINT('Ctrl Pts',(6.71586810234351,0.667974015272807,5.12771890448726));
#9055=CARTESIAN_POINT('Ctrl Pts',(6.71754218374966,0.676993827699967,5.19256731455862));
#9056=CARTESIAN_POINT('Ctrl Pts',(6.72057460952299,0.679835899888414,5.26655099041801));
#9057=CARTESIAN_POINT('Ctrl Pts',(6.73215258919641,0.666622431758416,5.39385244351734));
#9058=CARTESIAN_POINT('Ctrl Pts',(6.74808267646998,0.597703234226131,5.60637135858773));
#9059=CARTESIAN_POINT('Ctrl Pts',(6.76865865045639,0.42187569508026,5.80093567049644));
#9060=CARTESIAN_POINT('Ctrl Pts',(6.78775275289436,0.18949258292913,5.90281901720052));
#9061=CARTESIAN_POINT('Ctrl Pts',(6.80728398696971,-0.0613342485858974,
5.93720923449836));
#9062=CARTESIAN_POINT('Ctrl Pts',(6.83135970851047,-0.373059821574549,5.84556085535134));
#9063=CARTESIAN_POINT('Ctrl Pts',(6.85923191629717,-0.620447637519185,5.56518912958432));
#9064=CARTESIAN_POINT('Ctrl Pts',(6.88587504766456,-0.688763467578774,5.216551997357));
#9065=CARTESIAN_POINT('Ctrl Pts',(6.91139566465253,-0.586858521375168,4.89242219675425));
#9066=CARTESIAN_POINT('Ctrl Pts',(6.93682192897835,-0.343119258487298,4.6571125514519));
#9067=CARTESIAN_POINT('Ctrl Pts',(6.96217719555826,-0.017670596412725,4.56737841010226));
#9068=CARTESIAN_POINT('Ctrl Pts',(6.98745330968432,0.310091855530511,4.64383222378311));
#9069=CARTESIAN_POINT('Ctrl Pts',(7.01055807494553,0.539755215825518,4.8488411700511));
#9070=CARTESIAN_POINT('Ctrl Pts',(7.03150987721236,0.648059883045342,5.10140557124907));
#9071=CARTESIAN_POINT('Ctrl Pts',(7.05660277782412,0.660088135117788,5.43135081654961));
#9072=CARTESIAN_POINT('Ctrl Pts',(7.08371253109927,0.471238232523407,5.75442284803613));
#9073=CARTESIAN_POINT('Ctrl Pts',(7.11281790701897,0.116492402038094,5.91178575585197));
#9074=CARTESIAN_POINT('Ctrl Pts',(7.13771330081894,-0.213583901535594,5.88567475580613));
#9075=CARTESIAN_POINT('Ctrl Pts',(7.15738807567549,-0.433075159347389,5.74259656511571));
#9076=CARTESIAN_POINT('Ctrl Pts',(7.17186233961118,-0.546637546600257,5.59321236996226));
#9077=CARTESIAN_POINT('Ctrl Pts',(7.18426142057677,-0.618429896637663,5.44955013009039));
#9078=CARTESIAN_POINT('Ctrl Pts',(7.20593925357481,-0.671404712921254,5.16944154295922));
#9079=CARTESIAN_POINT('Ctrl Pts',(7.23685805149232,-0.514056507473933,4.7720238817847));
#9080=CARTESIAN_POINT('Ctrl Pts',(7.27388829057188,-0.0511187931748622,
4.55109735415634));
#9081=CARTESIAN_POINT('Ctrl Pts',(7.31086361178906,0.437321455158784,4.70378519211358));
#9082=CARTESIAN_POINT('Ctrl Pts',(7.34779990172598,0.691641488782215,5.14718657589742));
#9083=CARTESIAN_POINT('Ctrl Pts',(7.38471185454084,0.576388219284925,5.64538232477128));
#9084=CARTESIAN_POINT('Ctrl Pts',(7.41546811917344,0.224145749390111,5.88350929405959));
#9085=CARTESIAN_POINT('Ctrl Pts',(7.44007339032313,-0.0991038282370662,
5.89369455116736));
#9086=CARTESIAN_POINT('Ctrl Pts',(7.46058115581319,-0.353046546940354,5.80465440934753));
#9087=CARTESIAN_POINT('Ctrl Pts',(7.48315729994566,-0.567747214692048,5.59423252752844));
#9088=CARTESIAN_POINT('Ctrl Pts',(7.50779960123253,-0.663810701459249,5.28055053342104));
#9089=CARTESIAN_POINT('Ctrl Pts',(7.52834941587818,-0.608816343721552,5.01257565766459));
#9090=CARTESIAN_POINT('Ctrl Pts',(7.54479896304165,-0.492201788139917,4.83323933395727));
#9091=CARTESIAN_POINT('Ctrl Pts',(7.56125874789373,-0.335011840659567,4.68763787379617));
#9092=CARTESIAN_POINT('Ctrl Pts',(7.58185937612452,-0.0800643356826357,
4.58819992347848));
#9093=CARTESIAN_POINT('Ctrl Pts',(7.61072436677918,0.302026124742895,4.63563761482126));
#9094=CARTESIAN_POINT('Ctrl Pts',(7.63759060214969,0.573543629548249,4.88843827187382));
#9095=CARTESIAN_POINT('Ctrl Pts',(7.66243418548257,0.656176634414132,5.20452875813442));
#9096=CARTESIAN_POINT('Ctrl Pts',(7.68731798929925,0.620672834689613,5.52907101102389));
#9097=CARTESIAN_POINT('Ctrl Pts',(7.7185008361451,0.351786215425856,5.86676654532321));
#9098=CARTESIAN_POINT('Ctrl Pts',(7.75291850276096,-0.119163757158855,5.93680388820774));
#9099=CARTESIAN_POINT('Ctrl Pts',(7.78431371344778,-0.487788664582144,5.73191159498108));
#9100=CARTESIAN_POINT('Ctrl Pts',(7.81266278264196,-0.671728137594293,5.39915542463631));
#9101=CARTESIAN_POINT('Ctrl Pts',(7.83399695974143,-0.655495509577423,5.11326864305501));
#9102=CARTESIAN_POINT('Ctrl Pts',(7.84824319365684,-0.582304862321808,4.94409375866328));
#9103=CARTESIAN_POINT('Ctrl Pts',(7.85537248762996,-0.534328882072017,4.8653541422696));
#9104=CARTESIAN_POINT('Ctrl Pts',(7.8625080462426,-0.475697660357833,4.79396953698449));
#9105=CARTESIAN_POINT('Ctrl Pts',(7.87361834107539,-0.369870381089617,4.69696159670125));
#9106=CARTESIAN_POINT('Ctrl Pts',(7.89508364408438,-0.120581127165717,4.56363681242408));
#9107=CARTESIAN_POINT('Ctrl Pts',(7.92380487431976,0.274740702833653,4.59333951805747));
#9108=CARTESIAN_POINT('Ctrl Pts',(7.95587209874155,0.596060666569318,4.88149726068058));
#9109=CARTESIAN_POINT('Ctrl Pts',(7.98485490982878,0.703850404186812,5.25458043203598));
#9110=CARTESIAN_POINT('Ctrl Pts',(8.01395674562579,0.596009128666447,5.63029687158413));
#9111=CARTESIAN_POINT('Ctrl Pts',(8.04318557856648,0.303669437197963,5.89183096604927));
#9112=CARTESIAN_POINT('Ctrl Pts',(8.07254379370764,-0.0847679250430139,
5.95827083698362));
#9113=CARTESIAN_POINT('Ctrl Pts',(8.10203585350491,-0.450682443971355,5.80715198412111));
#9114=CARTESIAN_POINT('Ctrl Pts',(8.13166487881109,-0.68123591985956,5.48308204769604));
#9115=CARTESIAN_POINT('Ctrl Pts',(8.16143417804738,-0.704196784100177,5.08412597468992));
#9116=CARTESIAN_POINT('Ctrl Pts',(8.19134657907665,-0.510502727194234,4.73239774783289));
#9117=CARTESIAN_POINT('Ctrl Pts',(8.22140471118437,-0.157680363027014,4.53663054946559));
#9118=CARTESIAN_POINT('Ctrl Pts',(8.25161091715579,0.247209806959665,4.55863531050862));
#9119=CARTESIAN_POINT('Ctrl Pts',(8.28196721226589,0.580007046161269,4.79380459237181));
#9120=CARTESIAN_POINT('Ctrl Pts',(8.31247546153882,0.737522986966818,5.17184248687906));
#9121=CARTESIAN_POINT('Ctrl Pts',(8.3431369636528,0.669452578237767,5.57779897785294));
#9122=CARTESIAN_POINT('Ctrl Pts',(8.37395338723204,0.394549325777573,5.88686270419447));
#9123=CARTESIAN_POINT('Ctrl Pts',(8.40492468218856,-0.00477288997479829,
6.00301968920375));
#9124=CARTESIAN_POINT('Ctrl Pts',(8.43086566271663,-0.339484126663846,5.90732172989766));
#9125=CARTESIAN_POINT('Ctrl Pts',(8.45169393946564,-0.547072218093633,5.73229404684569));
#9126=CARTESIAN_POINT('Ctrl Pts',(8.47141407618564,-0.69056376988887,5.51909409327636));
#9127=CARTESIAN_POINT('Ctrl Pts',(8.49528051079703,-0.754506655121167,5.20780227421841));
#9128=CARTESIAN_POINT('Ctrl Pts',(8.52334094921819,-0.645203605665545,4.85064301321389));
#9129=CARTESIAN_POINT('Ctrl Pts',(8.54917704999056,-0.39970756208167,4.60951445591631));
#9130=CARTESIAN_POINT('Ctrl Pts',(8.57275318463256,-0.107751104615898,4.507212319962));
#9131=CARTESIAN_POINT('Ctrl Pts',(8.60113510608758,0.2652008828398,4.51862276966196));
#9132=CARTESIAN_POINT('Ctrl Pts',(8.63678462905851,0.674063216653352,4.79397580501787));
#9133=CARTESIAN_POINT('Ctrl Pts',(8.67983312698351,0.808996095068133,5.37521245548929));
#9134=CARTESIAN_POINT('Ctrl Pts',(8.72314631206897,0.511438980015273,5.89547267476356));
#9135=CARTESIAN_POINT('Ctrl Pts',(8.76671889614431,-0.0645101499886897,
6.07612806192154));
#9136=CARTESIAN_POINT('Ctrl Pts',(8.8032403134946,-0.52050637307905,5.85824970323195));
#9137=CARTESIAN_POINT('Ctrl Pts',(8.8325806026404,-0.725222219240906,5.53197478069197));
#9138=CARTESIAN_POINT('Ctrl Pts',(8.86200208878909,-0.800401500077765,5.15246739538599));
#9139=CARTESIAN_POINT('Ctrl Pts',(8.89400332481794,-0.641019042589212,4.74014811866369));
#9140=CARTESIAN_POINT('Ctrl Pts',(8.92861674579342,-0.253623824855234,4.48900662534079));
#9141=CARTESIAN_POINT('Ctrl Pts',(8.95838394375014,0.14096968639971,4.45739530277337));
#9142=CARTESIAN_POINT('Ctrl Pts',(8.98949233523325,0.519678120112436,4.62614772615488));
#9143=CARTESIAN_POINT('Ctrl Pts',(9.02194827654078,0.773504466413702,4.98022549611561));
#9144=CARTESIAN_POINT('Ctrl Pts',(9.05576659670161,0.801241182054453,5.43359139583031));
#9145=CARTESIAN_POINT('Ctrl Pts',(9.08969328319026,0.582823669257135,5.83337236814146));
#9146=CARTESIAN_POINT('Ctrl Pts',(9.12372119491323,0.183995572608789,6.0564428736434));
#9147=CARTESIAN_POINT('Ctrl Pts',(9.15784898234373,-0.273721773698358,6.03306963582005));
#9148=CARTESIAN_POINT('Ctrl Pts',(9.19205946304498,-0.64990994575872,5.76909502946593));
#9149=CARTESIAN_POINT('Ctrl Pts',(9.22636972842826,-0.828492853046594,5.34432711727714));
#9150=CARTESIAN_POINT('Ctrl Pts',(9.26071770907781,-0.753605783690083,4.88862365787852));
#9151=CARTESIAN_POINT('Ctrl Pts',(9.29521525363159,-0.447059278266013,4.54166254803362));
#9152=CARTESIAN_POINT('Ctrl Pts',(9.32385029237493,-0.076279701533059,4.43278968651557));
#9153=CARTESIAN_POINT('Ctrl Pts',(9.34704014326617,0.221568143128904,4.47363161156646));
#9154=CARTESIAN_POINT('Ctrl Pts',(9.36968427093344,0.497170404037412,4.59457970634328));
#9155=CARTESIAN_POINT('Ctrl Pts',(9.39402695598823,0.705082520374241,4.82463961699335));
#9156=CARTESIAN_POINT('Ctrl Pts',(9.41282588021654,0.786411815723876,5.07581826482597));
#9157=CARTESIAN_POINT('Ctrl Pts',(9.42644889255394,0.801979646461018,5.22505406419157));
#9158=CARTESIAN_POINT('Ctrl Pts',(9.43026740530825,0.798586255767136,5.31688402203871));
#9159=CARTESIAN_POINT('Ctrl Pts',(9.43215588553443,0.787994469037129,5.3917373403362));
#9160=CARTESIAN_POINT('Ctrl Pts',(9.43462005636334,0.77613860227658,5.44667996217276));
#9161=CARTESIAN_POINT('Ctrl Pts',(9.43675115866262,0.76054929407017,5.50053294126675));
#9162=CARTESIAN_POINT('Ctrl Pts',(9.44075039513402,0.721790412703208,5.60601810317749));
#9163=CARTESIAN_POINT('Ctrl Pts',(9.44711962463945,0.636128021011656,5.75304946126482));
#9164=CARTESIAN_POINT('Ctrl Pts',(9.45539179372209,0.471989769111388,5.90978296204479));
#9165=CARTESIAN_POINT('Ctrl Pts',(9.46376143836203,0.270776729544522,6.01500122015827));
#9166=CARTESIAN_POINT('Ctrl Pts',(9.47209357577949,0.048287231388412,6.06019930129363));
#9167=CARTESIAN_POINT('Ctrl Pts',(9.48323123102129,-0.253737210486127,6.03638375835141));
#9168=CARTESIAN_POINT('Ctrl Pts',(9.49713889491815,-0.595891436056078,5.84933347763517));
#9169=CARTESIAN_POINT('Ctrl Pts',(9.51385076478022,-0.823899220520506,5.4399993249345));
#9170=CARTESIAN_POINT('Ctrl Pts',(9.53056720336839,-0.798968852716643,4.97220899366434));
#9171=CARTESIAN_POINT('Ctrl Pts',(9.54729162985791,-0.528727439187925,4.58909409304663));
#9172=CARTESIAN_POINT('Ctrl Pts',(9.56402480986213,-0.0957723892084128,
4.40913981479913));
#9173=CARTESIAN_POINT('Ctrl Pts',(9.58076647982355,0.366654087604734,4.48684308047902));
#9174=CARTESIAN_POINT('Ctrl Pts',(9.59750846260415,0.71671035870106,4.79943942469371));
#9175=CARTESIAN_POINT('Ctrl Pts',(9.60867719102009,0.803285765633916,5.09951966622228));
#9176=CARTESIAN_POINT('Ctrl Pts',(9.61425624009638,0.803306050539573,5.25020145011708));
#9177=CARTESIAN_POINT('Ctrl Pts',(6.55994469204049,0.719709328495781,5.24703997894806));
#9178=CARTESIAN_POINT('Ctrl Pts',(6.56494552765653,0.719691145920131,5.38210508200347));
#9179=CARTESIAN_POINT('Ctrl Pts',(6.57494016333875,0.642089168505731,5.65058609468785));
#9180=CARTESIAN_POINT('Ctrl Pts',(6.58989438616266,0.32941528595114,5.9296313569664));
#9181=CARTESIAN_POINT('Ctrl Pts',(6.60481477071411,-0.0827797453005289,
5.99886361370576));
#9182=CARTESIAN_POINT('Ctrl Pts',(6.61969980345594,-0.467619845512657,5.83844773036597));
#9183=CARTESIAN_POINT('Ctrl Pts',(6.63454965842308,-0.707639327219362,5.49857002500469));
#9184=CARTESIAN_POINT('Ctrl Pts',(6.64936061260475,-0.729495436544756,5.0840660001111));
#9185=CARTESIAN_POINT('Ctrl Pts',(6.66414030226907,-0.527844751315962,4.72224444577032));
#9186=CARTESIAN_POINT('Ctrl Pts',(6.67641810037933,-0.225796647591973,4.55722222010489));
#9187=CARTESIAN_POINT('Ctrl Pts',(6.68623494447203,0.0403746271135037,4.5362580751361));
#9188=CARTESIAN_POINT('Ctrl Pts',(6.69357256905876,0.236291461979514,4.57606849800983));
#9189=CARTESIAN_POINT('Ctrl Pts',(6.70093718034598,0.413303779793928,4.66864974641035));
#9190=CARTESIAN_POINT('Ctrl Pts',(6.70820868996388,0.557592736564421,4.80642809587619));
#9191=CARTESIAN_POINT('Ctrl Pts',(6.71380490830661,0.632807795501951,4.93556873282767));
#9192=CARTESIAN_POINT('Ctrl Pts',(6.71731244248601,0.666836920456702,5.02812885948168));
#9193=CARTESIAN_POINT('Ctrl Pts',(6.71917582310349,0.680406120596861,5.07513188532028));
#9194=CARTESIAN_POINT('Ctrl Pts',(6.72133213271133,0.6909093875254,5.1233938812218));
#9195=CARTESIAN_POINT('Ctrl Pts',(6.72306773259333,0.700241175081311,5.19054637990825));
#9196=CARTESIAN_POINT('Ctrl Pts',(6.72619261442483,0.703178325652587,5.2668476785023));
#9197=CARTESIAN_POINT('Ctrl Pts',(6.7381664251681,0.689514001675121,5.39852659753196));
#9198=CARTESIAN_POINT('Ctrl Pts',(6.75463925550615,0.618247264838858,5.61826960075177));
#9199=CARTESIAN_POINT('Ctrl Pts',(6.77590827674278,0.436470460186145,5.81941560675087));
#9200=CARTESIAN_POINT('Ctrl Pts',(6.79564326301645,0.196280809931693,5.9247163591309));
#9201=CARTESIAN_POINT('Ctrl Pts',(6.81582644522033,-0.0629302930494358,
5.96025522192144));
#9202=CARTESIAN_POINT('Ctrl Pts',(6.84069654900574,-0.38497400844017,5.86555713916006));
#9203=CARTESIAN_POINT('Ctrl Pts',(6.86947638412051,-0.640427331596973,5.57601421543896));
#9204=CARTESIAN_POINT('Ctrl Pts',(6.89697365083529,-0.710923798883682,5.21615884811777));
#9205=CARTESIAN_POINT('Ctrl Pts',(6.92329898795441,-0.605777386429107,4.88177837844538));
#9206=CARTESIAN_POINT('Ctrl Pts',(6.94951107797999,-0.354456178032768,4.63917675459059));
#9207=CARTESIAN_POINT('Ctrl Pts',(6.97563701108018,-0.0190898795841548,
4.54673256040166));
#9208=CARTESIAN_POINT('Ctrl Pts',(7.00166306815893,0.318420157020357,4.6254869521555));
#9209=CARTESIAN_POINT('Ctrl Pts',(7.02543388521809,0.554722542828515,4.83645416115326));
#9210=CARTESIAN_POINT('Ctrl Pts',(7.04697773806416,0.666084600719225,5.09617679024369));
#9211=CARTESIAN_POINT('Ctrl Pts',(7.07276315353201,0.678427725557665,5.43526847721852));
#9212=CARTESIAN_POINT('Ctrl Pts',(7.10058962059944,0.484472501752673,5.76690932949108));
#9213=CARTESIAN_POINT('Ctrl Pts',(7.13043692169364,0.120638399689201,5.92825455906627));
#9214=CARTESIAN_POINT('Ctrl Pts',(7.1559402685194,-0.217537459809761,5.90145833585114));
#9215=CARTESIAN_POINT('Ctrl Pts',(7.17606991375773,-0.442156866353605,5.75500273582888));
#9216=CARTESIAN_POINT('Ctrl Pts',(7.1908732639631,-0.55830610816236,5.60220615030058));
#9217=CARTESIAN_POINT('Ctrl Pts',(7.20354845498638,-0.631705810891337,5.45532626907927));
#9218=CARTESIAN_POINT('Ctrl Pts',(7.22569553162755,-0.685810607871027,5.1691057765553));
#9219=CARTESIAN_POINT('Ctrl Pts',(7.25723947880328,-0.525122526582691,4.7636055764722));
#9220=CARTESIAN_POINT('Ctrl Pts',(7.29495362238925,-0.053457135933399,4.53870854204931));
#9221=CARTESIAN_POINT('Ctrl Pts',(7.33254246780218,0.443142598581714,4.69413693222259));
#9222=CARTESIAN_POINT('Ctrl Pts',(7.37001978026861,0.701091243696442,5.14423427781829));
#9223=CARTESIAN_POINT('Ctrl Pts',(7.40739968824424,0.584157721738047,5.64880921553006));
#9224=CARTESIAN_POINT('Ctrl Pts',(7.43848048896546,0.228011772623945,5.88938664283398));
#9225=CARTESIAN_POINT('Ctrl Pts',(7.46331103237168,-0.0982454758707846,
5.89962806423389));
#9226=CARTESIAN_POINT('Ctrl Pts',(7.48398628613683,-0.354294590444537,5.80983193950292));
#9227=CARTESIAN_POINT('Ctrl Pts',(7.50671008387199,-0.570451156260486,5.59791253961241));
#9228=CARTESIAN_POINT('Ctrl Pts',(7.53148051029953,-0.667000675030891,5.28247942808214));
#9229=CARTESIAN_POINT('Ctrl Pts',(7.55211030997723,-0.61172699107091,5.01340213779963));
#9230=CARTESIAN_POINT('Ctrl Pts',(7.56860908294787,-0.494743373007304,4.8335093105102));
#9231=CARTESIAN_POINT('Ctrl Pts',(7.58510523358743,-0.337168872759663,4.68756299395369));
#9232=CARTESIAN_POINT('Ctrl Pts',(7.60572192687897,-0.0819019612031444,
4.58805237352457));
#9233=CARTESIAN_POINT('Ctrl Pts',(7.63458408889819,0.300170619986696,4.63555033917682));
#9234=CARTESIAN_POINT('Ctrl Pts',(7.66138943476793,0.571053603076512,4.88796924826266));
#9235=CARTESIAN_POINT('Ctrl Pts',(7.68614446458683,0.653366892065435,5.20295921197447));
#9236=CARTESIAN_POINT('Ctrl Pts',(7.71090979818012,0.617991353788974,5.52603673989692));
#9237=CARTESIAN_POINT('Ctrl Pts',(7.74189055099461,0.350623503322525,5.86154592695952));
#9238=CARTESIAN_POINT('Ctrl Pts',(7.77601859800523,-0.116495965826188,5.93082813098408));
#9239=CARTESIAN_POINT('Ctrl Pts',(7.80709414997369,-0.481412412605556,5.72789933690448));
#9240=CARTESIAN_POINT('Ctrl Pts',(7.83510698559819,-0.663163478596285,5.39892523906655));
#9241=CARTESIAN_POINT('Ctrl Pts',(7.85615485977222,-0.647079306054213,5.11675578479515));
#9242=CARTESIAN_POINT('Ctrl Pts',(7.87020459706828,-0.574886104874813,4.94990033899215));
#9243=CARTESIAN_POINT('Ctrl Pts',(7.87723312367712,-0.527583060020924,4.87226677612988));
#9244=CARTESIAN_POINT('Ctrl Pts',(7.88426540124521,-0.469793796464868,4.80191051673322));
#9245=CARTESIAN_POINT('Ctrl Pts',(7.89521047892777,-0.365529336701908,4.7063343213378));
#9246=CARTESIAN_POINT('Ctrl Pts',(7.91634048666751,-0.120063962380262,4.57508935662309));
#9247=CARTESIAN_POINT('Ctrl Pts',(7.94458071734118,0.268642859242054,4.60441791433467));
#9248=CARTESIAN_POINT('Ctrl Pts',(7.97605533596052,0.584027938453731,4.88737223927164));
#9249=CARTESIAN_POINT('Ctrl Pts',(8.00446254702578,0.689638060716412,5.2531749302134));
#9250=CARTESIAN_POINT('Ctrl Pts',(8.03295521872146,0.583958260807566,5.62109535966095));
#9251=CARTESIAN_POINT('Ctrl Pts',(8.06153860386915,0.297951770638925,5.87686527268886));
#9252=CARTESIAN_POINT('Ctrl Pts',(8.09021776831132,-0.0816004700383042,
5.94171985993802));
#9253=CARTESIAN_POINT('Ctrl Pts',(8.11899761019108,-0.438736741574054,5.7941606881638));
#9254=CARTESIAN_POINT('Ctrl Pts',(8.14788283876726,-0.66350439566471,5.47812772009615));
#9255=CARTESIAN_POINT('Ctrl Pts',(8.17687795851733,-0.6858207744463,5.08946678694388));
#9256=CARTESIAN_POINT('Ctrl Pts',(8.20598727446933,-0.497249207778955,4.74714184053921));
#9257=CARTESIAN_POINT('Ctrl Pts',(8.23521486961617,-0.154093127286878,4.55679071733693));
#9258=CARTESIAN_POINT('Ctrl Pts',(8.26456461818433,0.239380388009074,4.57821827016813));
#9259=CARTESIAN_POINT('Ctrl Pts',(8.29404014876887,0.562549974717286,4.80663318942082));
#9260=CARTESIAN_POINT('Ctrl Pts',(8.32364486518472,0.715391021033525,5.17354565176085));
#9261=CARTESIAN_POINT('Ctrl Pts',(8.35338192623768,0.649330974858417,5.56731319891309));
#9262=CARTESIAN_POINT('Ctrl Pts',(8.38325424070601,0.382790348017333,5.86693311075399));
#9263=CARTESIAN_POINT('Ctrl Pts',(8.41326446409716,-0.00419505000370753,
5.97947359705855));
#9264=CARTESIAN_POINT('Ctrl Pts',(8.43838990507217,-0.328427739096548,5.88675138216907));
#9265=CARTESIAN_POINT('Ctrl Pts',(8.45856147729175,-0.529480619639225,5.71722997945441));
#9266=CARTESIAN_POINT('Ctrl Pts',(8.47765754585014,-0.668434606896997,5.5107649981822));
#9267=CARTESIAN_POINT('Ctrl Pts',(8.50076123794206,-0.730336170493974,5.20937619755011));
#9268=CARTESIAN_POINT('Ctrl Pts',(8.52792461605616,-0.624513035959022,4.86362366838459));
#9269=CARTESIAN_POINT('Ctrl Pts',(8.5529308052989,-0.386883838373545,4.6302289824672));
#9270=CARTESIAN_POINT('Ctrl Pts',(8.57574894485481,-0.104298108040022,4.53121501380808));
#9271=CARTESIAN_POINT('Ctrl Pts',(8.6032187287894,0.256675810750089,4.54226136093568));
#9272=CARTESIAN_POINT('Ctrl Pts',(8.63772155686955,0.652405168310869,4.80876975888547));
#9273=CARTESIAN_POINT('Ctrl Pts',(8.67939097890975,0.783030401351032,5.37140034010679));
#9274=CARTESIAN_POINT('Ctrl Pts',(8.72132656843746,0.49495090614558,5.87513455402037));
#9275=CARTESIAN_POINT('Ctrl Pts',(8.76352759225084,-0.0628635021467805,
6.05013777316939));
#9276=CARTESIAN_POINT('Ctrl Pts',(8.79891493140875,-0.504716359285686,5.83905645697925));
#9277=CARTESIAN_POINT('Ctrl Pts',(8.82735545219243,-0.703159459402567,5.5227896978014));
#9278=CARTESIAN_POINT('Ctrl Pts',(8.85588259535385,-0.776061781005718,5.15482469233793));
#9279=CARTESIAN_POINT('Ctrl Pts',(8.88692644387892,-0.621492770362474,4.75483748689365));
#9280=CARTESIAN_POINT('Ctrl Pts',(8.92052297991862,-0.245496738926199,4.51104937209089));
#9281=CARTESIAN_POINT('Ctrl Pts',(8.94943095663315,0.137693585331708,4.48033145317999));
#9282=CARTESIAN_POINT('Ctrl Pts',(8.97965767299615,0.505669735297425,4.64426980471776));
#9283=CARTESIAN_POINT('Ctrl Pts',(9.01121604967911,0.752482582266742,4.98850418901732));
#9284=CARTESIAN_POINT('Ctrl Pts',(9.04412144632782,0.779510405814253,5.42959222113123));
#9285=CARTESIAN_POINT('Ctrl Pts',(9.07715711994043,0.566889248726445,5.81885947968755));
#9286=CARTESIAN_POINT('Ctrl Pts',(9.11031735538565,0.178292209075846,6.0362617860296));
#9287=CARTESIAN_POINT('Ctrl Pts',(9.14360253722173,-0.268079437778697,6.01351727669282));
#9288=CARTESIAN_POINT('Ctrl Pts',(9.17699734546285,-0.635285771434068,5.75590592911153));
#9289=CARTESIAN_POINT('Ctrl Pts',(9.21051983173094,-0.809796215592389,5.34095865996421));
#9290=CARTESIAN_POINT('Ctrl Pts',(9.24411094986739,-0.736619369561702,4.89534022537719));
#9291=CARTESIAN_POINT('Ctrl Pts',(9.27788074499435,-0.436616793358521,4.55570108560577));
#9292=CARTESIAN_POINT('Ctrl Pts',(9.30594116368128,-0.0733420592947115,
4.44897069772665));
#9293=CARTESIAN_POINT('Ctrl Pts',(9.328680473888,0.218704827060702,4.48901682699427));
#9294=CARTESIAN_POINT('Ctrl Pts',(9.35089495840618,0.489065381509997,4.60762593183536));
#9295=CARTESIAN_POINT('Ctrl Pts',(9.37480209610635,0.693278005812641,4.83358316838714));
#9296=CARTESIAN_POINT('Ctrl Pts',(9.39327740184756,0.773205179450414,5.08031011736591));
#9297=CARTESIAN_POINT('Ctrl Pts',(9.40667901531909,0.788514168138214,5.22730031946394));
#9298=CARTESIAN_POINT('Ctrl Pts',(9.41035265957923,0.785191918284243,5.31605807341251));
#9299=CARTESIAN_POINT('Ctrl Pts',(9.41223809751033,0.774762970480976,5.39019446309586));
#9300=CARTESIAN_POINT('Ctrl Pts',(9.4146591021466,0.763068583364469,5.44423938068532));
#9301=CARTESIAN_POINT('Ctrl Pts',(9.4167523666832,0.747778571803171,5.49710428778674));
#9302=CARTESIAN_POINT('Ctrl Pts',(9.42068446598339,0.709658392601865,5.60083098220104));
#9303=CARTESIAN_POINT('Ctrl Pts',(9.42695148511213,0.625399217361514,5.74546397737963));
#9304=CARTESIAN_POINT('Ctrl Pts',(9.4350913459169,0.463897848898915,5.89967743034001));
#9305=CARTESIAN_POINT('Ctrl Pts',(9.44332988824765,0.265871334396363,6.00323600320908));
#9306=CARTESIAN_POINT('Ctrl Pts',(9.45153347644623,0.0468430344411857,6.04773546710682));
#9307=CARTESIAN_POINT('Ctrl Pts',(9.46250188685132,-0.250556076226033,6.02429177474909));
#9308=CARTESIAN_POINT('Ctrl Pts',(9.47620737800529,-0.587650060167328,5.84004639330421));
#9309=CARTESIAN_POINT('Ctrl Pts',(9.49268366719886,-0.81241635296479,5.43659555942134));
#9310=CARTESIAN_POINT('Ctrl Pts',(9.50917374900608,-0.787865415172378,4.9752477474741));
#9311=CARTESIAN_POINT('Ctrl Pts',(9.52568233488031,-0.521201295938573,4.59717415541696));
#9312=CARTESIAN_POINT('Ctrl Pts',(9.5422061736552,-0.0937383220535699,4.41946428983354));
#9313=CARTESIAN_POINT('Ctrl Pts',(9.55874735915243,0.363109547604185,4.49620059730279));
#9314=CARTESIAN_POINT('Ctrl Pts',(9.57529830568314,0.709172657538417,4.80516325810888));
#9315=CARTESIAN_POINT('Ctrl Pts',(9.58634758255215,0.794862864598598,5.10196837702893));
#9316=CARTESIAN_POINT('Ctrl Pts',(9.59186670251247,0.79488293160754,5.25103156499837));
#9317=CARTESIAN_POINT('',(6.55994469204049,0.719709328495781,5.24703997894806));
#9318=CARTESIAN_POINT('Origin',(6.48,0.72,5.25));
#9319=CARTESIAN_POINT('',(9.59186670251247,0.79488293160754,5.25103156499837));
#9320=CARTESIAN_POINT('Ctrl Pts',(6.55994469204049,0.719709328495781,5.24703997894806));
#9321=CARTESIAN_POINT('Ctrl Pts',(6.56494552765653,0.719691145920131,5.38210508200347));
#9322=CARTESIAN_POINT('Ctrl Pts',(6.57494016333875,0.642089168505731,5.65058609468785));
#9323=CARTESIAN_POINT('Ctrl Pts',(6.58989438616266,0.32941528595114,5.9296313569664));
#9324=CARTESIAN_POINT('Ctrl Pts',(6.60481477071411,-0.0827797453005289,
5.99886361370576));
#9325=CARTESIAN_POINT('Ctrl Pts',(6.61969980345594,-0.467619845512657,5.83844773036597));
#9326=CARTESIAN_POINT('Ctrl Pts',(6.63454965842308,-0.707639327219362,5.49857002500469));
#9327=CARTESIAN_POINT('Ctrl Pts',(6.64936061260475,-0.729495436544756,5.0840660001111));
#9328=CARTESIAN_POINT('Ctrl Pts',(6.66414030226907,-0.527844751315962,4.72224444577032));
#9329=CARTESIAN_POINT('Ctrl Pts',(6.67641810037933,-0.225796647591973,4.55722222010489));
#9330=CARTESIAN_POINT('Ctrl Pts',(6.68623494447203,0.0403746271135037,4.5362580751361));
#9331=CARTESIAN_POINT('Ctrl Pts',(6.69357256905876,0.236291461979514,4.57606849800983));
#9332=CARTESIAN_POINT('Ctrl Pts',(6.70093718034598,0.413303779793928,4.66864974641035));
#9333=CARTESIAN_POINT('Ctrl Pts',(6.70820868996388,0.557592736564421,4.80642809587619));
#9334=CARTESIAN_POINT('Ctrl Pts',(6.71380490830661,0.632807795501951,4.93556873282767));
#9335=CARTESIAN_POINT('Ctrl Pts',(6.71731244248601,0.666836920456702,5.02812885948168));
#9336=CARTESIAN_POINT('Ctrl Pts',(6.71917582310349,0.680406120596861,5.07513188532028));
#9337=CARTESIAN_POINT('Ctrl Pts',(6.72133213271133,0.6909093875254,5.1233938812218));
#9338=CARTESIAN_POINT('Ctrl Pts',(6.72306773259333,0.700241175081311,5.19054637990825));
#9339=CARTESIAN_POINT('Ctrl Pts',(6.72619261442483,0.703178325652587,5.2668476785023));
#9340=CARTESIAN_POINT('Ctrl Pts',(6.7381664251681,0.689514001675121,5.39852659753196));
#9341=CARTESIAN_POINT('Ctrl Pts',(6.75463925550615,0.618247264838858,5.61826960075177));
#9342=CARTESIAN_POINT('Ctrl Pts',(6.77590827674278,0.436470460186145,5.81941560675087));
#9343=CARTESIAN_POINT('Ctrl Pts',(6.79564326301645,0.196280809931693,5.9247163591309));
#9344=CARTESIAN_POINT('Ctrl Pts',(6.81582644522033,-0.0629302930494358,
5.96025522192144));
#9345=CARTESIAN_POINT('Ctrl Pts',(6.84069654900574,-0.38497400844017,5.86555713916006));
#9346=CARTESIAN_POINT('Ctrl Pts',(6.86947638412051,-0.640427331596973,5.57601421543896));
#9347=CARTESIAN_POINT('Ctrl Pts',(6.89697365083529,-0.710923798883682,5.21615884811777));
#9348=CARTESIAN_POINT('Ctrl Pts',(6.92329898795441,-0.605777386429107,4.88177837844538));
#9349=CARTESIAN_POINT('Ctrl Pts',(6.94951107797999,-0.354456178032768,4.63917675459059));
#9350=CARTESIAN_POINT('Ctrl Pts',(6.97563701108018,-0.0190898795841548,
4.54673256040166));
#9351=CARTESIAN_POINT('Ctrl Pts',(7.00166306815893,0.318420157020357,4.6254869521555));
#9352=CARTESIAN_POINT('Ctrl Pts',(7.02543388521809,0.554722542828515,4.83645416115326));
#9353=CARTESIAN_POINT('Ctrl Pts',(7.04697773806416,0.666084600719225,5.09617679024369));
#9354=CARTESIAN_POINT('Ctrl Pts',(7.07276315353201,0.678427725557665,5.43526847721852));
#9355=CARTESIAN_POINT('Ctrl Pts',(7.10058962059944,0.484472501752673,5.76690932949108));
#9356=CARTESIAN_POINT('Ctrl Pts',(7.13043692169364,0.120638399689201,5.92825455906627));
#9357=CARTESIAN_POINT('Ctrl Pts',(7.1559402685194,-0.217537459809761,5.90145833585114));
#9358=CARTESIAN_POINT('Ctrl Pts',(7.17606991375773,-0.442156866353605,5.75500273582888));
#9359=CARTESIAN_POINT('Ctrl Pts',(7.1908732639631,-0.55830610816236,5.60220615030058));
#9360=CARTESIAN_POINT('Ctrl Pts',(7.20354845498638,-0.631705810891337,5.45532626907927));
#9361=CARTESIAN_POINT('Ctrl Pts',(7.22569553162755,-0.685810607871027,5.1691057765553));
#9362=CARTESIAN_POINT('Ctrl Pts',(7.25723947880328,-0.525122526582691,4.7636055764722));
#9363=CARTESIAN_POINT('Ctrl Pts',(7.29495362238925,-0.053457135933399,4.53870854204931));
#9364=CARTESIAN_POINT('Ctrl Pts',(7.33254246780218,0.443142598581714,4.69413693222259));
#9365=CARTESIAN_POINT('Ctrl Pts',(7.37001978026861,0.701091243696442,5.14423427781829));
#9366=CARTESIAN_POINT('Ctrl Pts',(7.40739968824424,0.584157721738047,5.64880921553006));
#9367=CARTESIAN_POINT('Ctrl Pts',(7.43848048896546,0.228011772623945,5.88938664283398));
#9368=CARTESIAN_POINT('Ctrl Pts',(7.46331103237168,-0.0982454758707846,
5.89962806423389));
#9369=CARTESIAN_POINT('Ctrl Pts',(7.48398628613683,-0.354294590444537,5.80983193950292));
#9370=CARTESIAN_POINT('Ctrl Pts',(7.50671008387199,-0.570451156260486,5.59791253961241));
#9371=CARTESIAN_POINT('Ctrl Pts',(7.53148051029953,-0.667000675030891,5.28247942808214));
#9372=CARTESIAN_POINT('Ctrl Pts',(7.55211030997723,-0.61172699107091,5.01340213779963));
#9373=CARTESIAN_POINT('Ctrl Pts',(7.56860908294787,-0.494743373007304,4.8335093105102));
#9374=CARTESIAN_POINT('Ctrl Pts',(7.58510523358743,-0.337168872759663,4.68756299395369));
#9375=CARTESIAN_POINT('Ctrl Pts',(7.60572192687897,-0.0819019612031444,
4.58805237352457));
#9376=CARTESIAN_POINT('Ctrl Pts',(7.63458408889819,0.300170619986696,4.63555033917682));
#9377=CARTESIAN_POINT('Ctrl Pts',(7.66138943476793,0.571053603076512,4.88796924826266));
#9378=CARTESIAN_POINT('Ctrl Pts',(7.68614446458683,0.653366892065435,5.20295921197447));
#9379=CARTESIAN_POINT('Ctrl Pts',(7.71090979818012,0.617991353788974,5.52603673989692));
#9380=CARTESIAN_POINT('Ctrl Pts',(7.74189055099461,0.350623503322525,5.86154592695952));
#9381=CARTESIAN_POINT('Ctrl Pts',(7.77601859800523,-0.116495965826188,5.93082813098408));
#9382=CARTESIAN_POINT('Ctrl Pts',(7.80709414997369,-0.481412412605556,5.72789933690448));
#9383=CARTESIAN_POINT('Ctrl Pts',(7.83510698559819,-0.663163478596285,5.39892523906655));
#9384=CARTESIAN_POINT('Ctrl Pts',(7.85615485977222,-0.647079306054213,5.11675578479515));
#9385=CARTESIAN_POINT('Ctrl Pts',(7.87020459706828,-0.574886104874813,4.94990033899215));
#9386=CARTESIAN_POINT('Ctrl Pts',(7.87723312367712,-0.527583060020924,4.87226677612988));
#9387=CARTESIAN_POINT('Ctrl Pts',(7.88426540124521,-0.469793796464868,4.80191051673322));
#9388=CARTESIAN_POINT('Ctrl Pts',(7.89521047892777,-0.365529336701908,4.7063343213378));
#9389=CARTESIAN_POINT('Ctrl Pts',(7.91634048666751,-0.120063962380262,4.57508935662309));
#9390=CARTESIAN_POINT('Ctrl Pts',(7.94458071734118,0.268642859242054,4.60441791433467));
#9391=CARTESIAN_POINT('Ctrl Pts',(7.97605533596052,0.584027938453731,4.88737223927164));
#9392=CARTESIAN_POINT('Ctrl Pts',(8.00446254702578,0.689638060716412,5.2531749302134));
#9393=CARTESIAN_POINT('Ctrl Pts',(8.03295521872146,0.583958260807566,5.62109535966095));
#9394=CARTESIAN_POINT('Ctrl Pts',(8.06153860386915,0.297951770638925,5.87686527268886));
#9395=CARTESIAN_POINT('Ctrl Pts',(8.09021776831132,-0.0816004700383042,
5.94171985993802));
#9396=CARTESIAN_POINT('Ctrl Pts',(8.11899761019108,-0.438736741574054,5.7941606881638));
#9397=CARTESIAN_POINT('Ctrl Pts',(8.14788283876726,-0.66350439566471,5.47812772009615));
#9398=CARTESIAN_POINT('Ctrl Pts',(8.17687795851733,-0.6858207744463,5.08946678694388));
#9399=CARTESIAN_POINT('Ctrl Pts',(8.20598727446933,-0.497249207778955,4.74714184053921));
#9400=CARTESIAN_POINT('Ctrl Pts',(8.23521486961617,-0.154093127286878,4.55679071733693));
#9401=CARTESIAN_POINT('Ctrl Pts',(8.26456461818433,0.239380388009074,4.57821827016813));
#9402=CARTESIAN_POINT('Ctrl Pts',(8.29404014876887,0.562549974717286,4.80663318942082));
#9403=CARTESIAN_POINT('Ctrl Pts',(8.32364486518472,0.715391021033525,5.17354565176085));
#9404=CARTESIAN_POINT('Ctrl Pts',(8.35338192623768,0.649330974858417,5.56731319891309));
#9405=CARTESIAN_POINT('Ctrl Pts',(8.38325424070601,0.382790348017333,5.86693311075399));
#9406=CARTESIAN_POINT('Ctrl Pts',(8.41326446409716,-0.00419505000370753,
5.97947359705855));
#9407=CARTESIAN_POINT('Ctrl Pts',(8.43838990507217,-0.328427739096548,5.88675138216907));
#9408=CARTESIAN_POINT('Ctrl Pts',(8.45856147729175,-0.529480619639225,5.71722997945441));
#9409=CARTESIAN_POINT('Ctrl Pts',(8.47765754585014,-0.668434606896997,5.5107649981822));
#9410=CARTESIAN_POINT('Ctrl Pts',(8.50076123794206,-0.730336170493974,5.20937619755011));
#9411=CARTESIAN_POINT('Ctrl Pts',(8.52792461605616,-0.624513035959022,4.86362366838459));
#9412=CARTESIAN_POINT('Ctrl Pts',(8.5529308052989,-0.386883838373545,4.6302289824672));
#9413=CARTESIAN_POINT('Ctrl Pts',(8.57574894485481,-0.104298108040022,4.53121501380808));
#9414=CARTESIAN_POINT('Ctrl Pts',(8.6032187287894,0.256675810750089,4.54226136093568));
#9415=CARTESIAN_POINT('Ctrl Pts',(8.63772155686955,0.652405168310869,4.80876975888547));
#9416=CARTESIAN_POINT('Ctrl Pts',(8.67939097890975,0.783030401351032,5.37140034010679));
#9417=CARTESIAN_POINT('Ctrl Pts',(8.72132656843746,0.49495090614558,5.87513455402037));
#9418=CARTESIAN_POINT('Ctrl Pts',(8.76352759225084,-0.0628635021467805,
6.05013777316939));
#9419=CARTESIAN_POINT('Ctrl Pts',(8.79891493140875,-0.504716359285686,5.83905645697925));
#9420=CARTESIAN_POINT('Ctrl Pts',(8.82735545219243,-0.703159459402567,5.5227896978014));
#9421=CARTESIAN_POINT('Ctrl Pts',(8.85588259535385,-0.776061781005718,5.15482469233793));
#9422=CARTESIAN_POINT('Ctrl Pts',(8.88692644387892,-0.621492770362474,4.75483748689365));
#9423=CARTESIAN_POINT('Ctrl Pts',(8.92052297991862,-0.245496738926199,4.51104937209089));
#9424=CARTESIAN_POINT('Ctrl Pts',(8.94943095663315,0.137693585331708,4.48033145317999));
#9425=CARTESIAN_POINT('Ctrl Pts',(8.97965767299615,0.505669735297425,4.64426980471776));
#9426=CARTESIAN_POINT('Ctrl Pts',(9.01121604967911,0.752482582266742,4.98850418901732));
#9427=CARTESIAN_POINT('Ctrl Pts',(9.04412144632782,0.779510405814253,5.42959222113123));
#9428=CARTESIAN_POINT('Ctrl Pts',(9.07715711994043,0.566889248726445,5.81885947968755));
#9429=CARTESIAN_POINT('Ctrl Pts',(9.11031735538565,0.178292209075846,6.0362617860296));
#9430=CARTESIAN_POINT('Ctrl Pts',(9.14360253722173,-0.268079437778697,6.01351727669282));
#9431=CARTESIAN_POINT('Ctrl Pts',(9.17699734546285,-0.635285771434068,5.75590592911153));
#9432=CARTESIAN_POINT('Ctrl Pts',(9.21051983173094,-0.809796215592389,5.34095865996421));
#9433=CARTESIAN_POINT('Ctrl Pts',(9.24411094986739,-0.736619369561702,4.89534022537719));
#9434=CARTESIAN_POINT('Ctrl Pts',(9.27788074499435,-0.436616793358521,4.55570108560577));
#9435=CARTESIAN_POINT('Ctrl Pts',(9.30594116368128,-0.0733420592947115,
4.44897069772665));
#9436=CARTESIAN_POINT('Ctrl Pts',(9.328680473888,0.218704827060702,4.48901682699427));
#9437=CARTESIAN_POINT('Ctrl Pts',(9.35089495840618,0.489065381509997,4.60762593183536));
#9438=CARTESIAN_POINT('Ctrl Pts',(9.37480209610635,0.693278005812641,4.83358316838714));
#9439=CARTESIAN_POINT('Ctrl Pts',(9.39327740184756,0.773205179450414,5.08031011736591));
#9440=CARTESIAN_POINT('Ctrl Pts',(9.40667901531909,0.788514168138214,5.22730031946394));
#9441=CARTESIAN_POINT('Ctrl Pts',(9.41035265957923,0.785191918284243,5.31605807341251));
#9442=CARTESIAN_POINT('Ctrl Pts',(9.41223809751033,0.774762970480976,5.39019446309586));
#9443=CARTESIAN_POINT('Ctrl Pts',(9.4146591021466,0.763068583364469,5.44423938068532));
#9444=CARTESIAN_POINT('Ctrl Pts',(9.4167523666832,0.747778571803171,5.49710428778674));
#9445=CARTESIAN_POINT('Ctrl Pts',(9.42068446598339,0.709658392601865,5.60083098220104));
#9446=CARTESIAN_POINT('Ctrl Pts',(9.42695148511213,0.625399217361514,5.74546397737963));
#9447=CARTESIAN_POINT('Ctrl Pts',(9.4350913459169,0.463897848898915,5.89967743034001));
#9448=CARTESIAN_POINT('Ctrl Pts',(9.44332988824765,0.265871334396363,6.00323600320908));
#9449=CARTESIAN_POINT('Ctrl Pts',(9.45153347644623,0.0468430344411857,6.04773546710682));
#9450=CARTESIAN_POINT('Ctrl Pts',(9.46250188685132,-0.250556076226033,6.02429177474909));
#9451=CARTESIAN_POINT('Ctrl Pts',(9.47620737800529,-0.587650060167328,5.84004639330421));
#9452=CARTESIAN_POINT('Ctrl Pts',(9.49268366719886,-0.81241635296479,5.43659555942134));
#9453=CARTESIAN_POINT('Ctrl Pts',(9.50917374900608,-0.787865415172378,4.9752477474741));
#9454=CARTESIAN_POINT('Ctrl Pts',(9.52568233488031,-0.521201295938573,4.59717415541696));
#9455=CARTESIAN_POINT('Ctrl Pts',(9.5422061736552,-0.0937383220535699,4.41946428983354));
#9456=CARTESIAN_POINT('Ctrl Pts',(9.55874735915243,0.363109547604185,4.49620059730279));
#9457=CARTESIAN_POINT('Ctrl Pts',(9.57529830568314,0.709172657538417,4.80516325810888));
#9458=CARTESIAN_POINT('Ctrl Pts',(9.58634758255215,0.794862864598598,5.10196837702893));
#9459=CARTESIAN_POINT('Ctrl Pts',(9.59186670251247,0.79488293160754,5.25103156499837));
#9460=CARTESIAN_POINT('Origin',(9.61999999999987,0.720000000000002,5.25));
#9461=CARTESIAN_POINT('Origin',(9.61999999999987,0.720000000000002,5.25));
#9462=CARTESIAN_POINT('Origin',(6.48,0.72,5.25));
#10976=UNCERTAINTY_MEASURE_WITH_UNIT(LENGTH_MEASURE(0.001),#11036,
'DISTANCE_ACCURACY_VALUE',
'Maximum model space distance between geometric entities at asserted c
onnectivities');
#11002=UNCERTAINTY_MEASURE_WITH_UNIT(LENGTH_MEASURE(0.001),#11036,
'DISTANCE_ACCURACY_VALUE',
'Maximum model space distance between geometric entities at asserted c
onnectivities');
#11009=(
GEOMETRIC_REPRESENTATION_CONTEXT(3)
GLOBAL_UNCERTAINTY_ASSIGNED_CONTEXT((#10976))
GLOBAL_UNIT_ASSIGNED_CONTEXT((#11036,#11038,#11039))
REPRESENTATION_CONTEXT('','3D')
);
#11035=(
GEOMETRIC_REPRESENTATION_CONTEXT(3)
GLOBAL_UNCERTAINTY_ASSIGNED_CONTEXT((#11002))
GLOBAL_UNIT_ASSIGNED_CONTEXT((#11036,#11038,#11039))
REPRESENTATION_CONTEXT('','3D')
);
#11036=(
LENGTH_UNIT()
NAMED_UNIT(*)
SI_UNIT(.CENTI.,.METRE.)
);
#11038=(
NAMED_UNIT(*)
PLANE_ANGLE_UNIT()
SI_UNIT($,.RADIAN.)
);
#11039=(
NAMED_UNIT(*)
SI_UNIT($,.STERADIAN.)
SOLID_ANGLE_UNIT()
);
#11046=SHAPE_DEFINITION_REPRESENTATION(#11078,#11159);
#11078=PRODUCT_DEFINITION_SHAPE('',$,#11192);
#11159=SHAPE_REPRESENTATION('',(#5143),#11009);
#11185=PRODUCT_DEFINITION_CONTEXT('part definition',#11283,'design');
#11192=PRODUCT_DEFINITION('Installed follower spring',
'Installed follower spring',#11224,#11185);
#11224=PRODUCT_DEFINITION_FORMATION('',$,#11291);
#11283=APPLICATION_CONTEXT(
'Core Data for Automotive Mechanical Design Process');
#11284=PRODUCT_CONTEXT('part definition',#11283,'mechanical');
#11291=PRODUCT('Installed follower spring','Installed follower spring',
'Installed follower spring',(#11284));
#11380=COLOUR_RGB('Grey',0.48,0.52,0.57);
#11381=FILL_AREA_STYLE_COLOUR('',#11380);
#11382=FILL_AREA_STYLE('',(#11381));
#11383=SURFACE_STYLE_FILL_AREA(#11382);
#11384=SURFACE_SIDE_STYLE('',(#11383));
#11385=SURFACE_STYLE_USAGE(.BOTH.,#11384);
#11386=PRESENTATION_STYLE_ASSIGNMENT((#11385));
ENDSEC;
END-ISO-10303-21;
